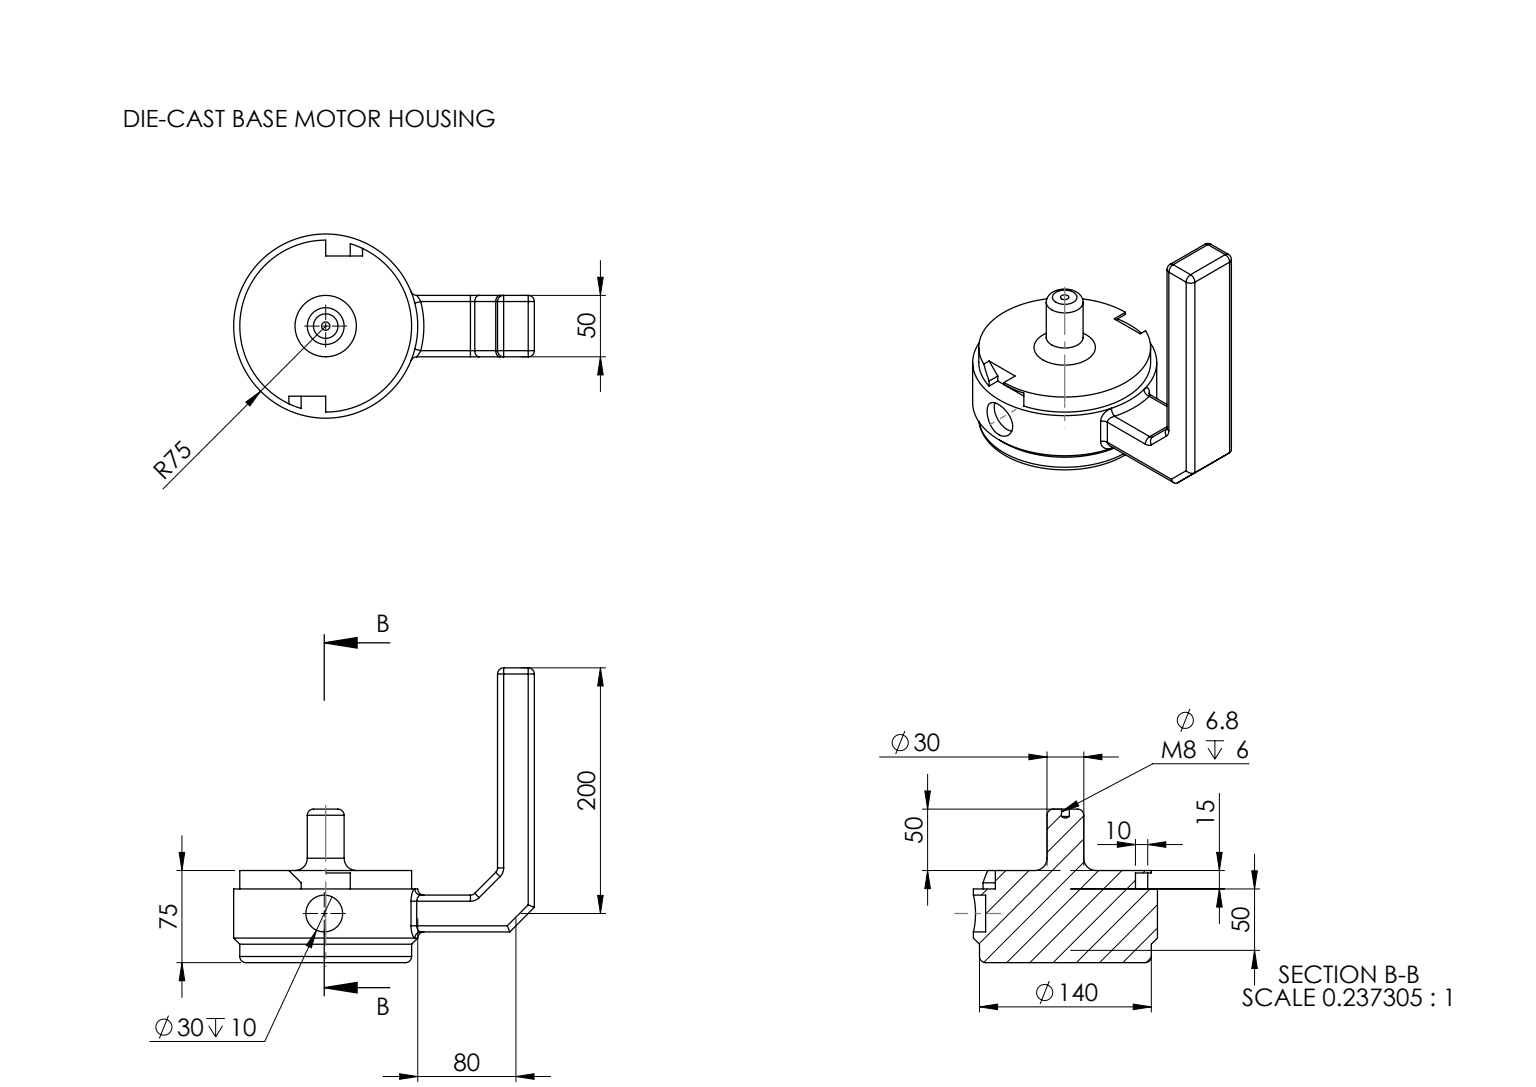
ISO-10303-21;
HEADER;
FILE_DESCRIPTION (('STEP AP214'),
    '1' );
FILE_NAME ('Die-Cast Base Motor Housing.step',
    '2026-10-08T14:59:03',
    ( '' ),
    ( '' ),
    'SwSTEP 2.0',
    'SolidWorks 2026',
    '' );
FILE_SCHEMA (( 'AUTOMOTIVE_DESIGN' ));
ENDSEC;

DATA;
#3=CARTESIAN_POINT ( 'NONE',  ( 71.93323519045090109, 49.64954395535312415, 21.22984507177767100 ) ) ;
#9=MECHANICAL_DESIGN_GEOMETRIC_PRESENTATION_REPRESENTATION('',(#5399),#3796);
#10=CARTESIAN_POINT ( 'NONE',  ( 1.836970198721029589E-15, 110.0000000000000000, 15.00000000000000000 ) ) ;
#18=CYLINDRICAL_SURFACE ( 'NONE', #1272, 5.000000000000001776 ) ;
#31=CARTESIAN_POINT ( 'NONE',  ( 74.19588822391826000, 40.66783446091307042, -24.95803700703555350 ) ) ;
#36=CARTESIAN_POINT ( 'NONE',  ( 77.29209776116614705, 15.00000000000009059, -20.32449628861697377 ) ) ;
#44=VERTEX_POINT ( 'NONE', #11902 ) ;
#50=CARTESIAN_POINT ( 'NONE',  ( 170.0000000000011369, 35.00000000000004974, -19.99999999999999645 ) ) ;
#51=VERTEX_POINT ( 'NONE', #2763 ) ;
#52=ADVANCED_FACE ( 'NONE', ( #8078 ), #12195, .T. ) ;
#53=PLANE ( 'NONE',  #708 ) ;
#58=VECTOR ( 'NONE', #5099, 1000.000000000000000 ) ;
#61=ADVANCED_FACE ( 'NONE', ( #9422 ), #904, .T. ) ;
#63=ADVANCED_FACE ( 'NONE', ( #7151 ), #4694, .T. ) ;
#64=CARTESIAN_POINT ( 'NONE',  ( -5.632982942078911925, 15.66369320862007264, 74.78974241430267966 ) ) ;
#75=CARTESIAN_POINT ( 'NONE',  ( 72.29554967163173274, 10.06394264408140771, 19.96827991394381030 ) ) ;
#79=AXIS2_PLACEMENT_3D ( 'NONE', #1491, #4293, #8024 ) ;
#81=CYLINDRICAL_SURFACE ( 'NONE', #3664, 5.000000000000000888 ) ;
#94=CARTESIAN_POINT ( 'NONE',  ( 74.77359728361332714, 42.68513822356444365, -24.22100760279283094 ) ) ;
#98=DIRECTION ( 'NONE',  ( 1.000000000000000000, 0.000000000000000000, -3.469446951953613203E-16 ) ) ;
#117=DIRECTION ( 'NONE',  ( 1.000000000000000000, -0.000000000000000000, 0.000000000000000000 ) ) ;
#121=ORIENTED_EDGE ( 'NONE', *, *, #6558, .F. ) ;
#123=DIRECTION ( 'NONE',  ( 1.000000000000000000, 0.000000000000000000, 0.000000000000000000 ) ) ;
#128=PLANE ( 'NONE',  #8446 ) ;
#131=DIRECTION ( 'NONE',  ( -1.000000000000000000, -1.387778780781444492E-15, 0.000000000000000000 ) ) ;
#134=CARTESIAN_POINT ( 'NONE',  ( 69.52686081652184669, 20.00000000000009237, -28.12499999999999645 ) ) ;
#137=CARTESIAN_POINT ( 'NONE',  ( 20.00000000000000000, 7.965803112215716020, -67.08203932499371547 ) ) ;
#141=ADVANCED_FACE ( 'NONE', ( #5767 ), #10055, .F. ) ;
#143=PLANE ( 'NONE',  #4255 ) ;
#149=DIRECTION ( 'NONE',  ( -0.000000000000000000, -0.000000000000000000, 1.000000000000000000 ) ) ;
#155=FILL_AREA_STYLE_COLOUR ( '', #11172 ) ;
#157=CARTESIAN_POINT ( 'NONE',  ( 70.81305327821827689, 40.84876555524851938, -24.93520811514266100 ) ) ;
#164=CARTESIAN_POINT ( 'NONE',  ( 76.56941542346943663, 15.25646994755911656, -21.58911091692574047 ) ) ;
#172=DIRECTION ( 'NONE',  ( 1.000000000000000000, 0.000000000000000000, 3.469446951953613203E-16 ) ) ;
#177=ORIENTED_EDGE ( 'NONE', *, *, #6032, .T. ) ;
#179=VECTOR ( 'NONE', #1966, 1000.000000000000000 ) ;
#192=ORIENTED_EDGE ( 'NONE', *, *, #11363, .T. ) ;
#194=CARTESIAN_POINT ( 'NONE',  ( 150.0000000000010800, 15.00000000000008882, 20.00000000000000000 ) ) ;
#201=CARTESIAN_POINT ( 'NONE',  ( 72.61843774138908714, 15.00000000000009059, 18.75000000000000355 ) ) ;
#202=CIRCLE ( 'NONE', #8371, 5.000000000000000888 ) ;
#203=ORIENTED_EDGE ( 'NONE', *, *, #11363, .F. ) ;
#206=VECTOR ( 'NONE', #5383, 1000.000000000000000 ) ;
#208=CARTESIAN_POINT ( 'NONE',  ( 13.11499952929491641, 34.60506461548092716, 73.84520852716261174 ) ) ;
#210=DIRECTION ( 'NONE',  ( -0.7071067811865503483, -0.7071067811865447972, -0.000000000000000000 ) ) ;
#211=DIRECTION ( 'NONE',  ( 0.000000000000000000, 1.000000000000000000, 0.000000000000000000 ) ) ;
#212=CARTESIAN_POINT ( 'NONE',  ( 0.000000000000000000, 10.00000000000017586, 0.000000000000000000 ) ) ;
#218=( LENGTH_UNIT ( ) NAMED_UNIT ( * ) SI_UNIT ( .MILLI., .METRE. ) );
#219=EDGE_CURVE ( 'NONE', #4313, #6757, #4559, .T. ) ;
#222=FACE_OUTER_BOUND ( 'NONE', #11804, .T. ) ;
#225=ADVANCED_FACE ( 'NONE', ( #3686 ), #6591, .F. ) ;
#229=CARTESIAN_POINT ( 'NONE',  ( 71.00672680945956472, 11.81742436800341345, -24.14780939829461204 ) ) ;
#234=AXIS2_PLACEMENT_3D ( 'NONE', #9468, #5745, #3808 ) ;
#250=VECTOR ( 'NONE', #7783, 1000.000000000000000 ) ;
#252=DIRECTION ( 'NONE',  ( -0.000000000000000000, 1.000000000000000000, -0.000000000000000000 ) ) ;
#254=CYLINDRICAL_SURFACE ( 'NONE', #5879, 5.000000000000000888 ) ;
#257=DIRECTION ( 'NONE',  ( -0.000000000000000000, -0.000000000000000000, 1.000000000000000000 ) ) ;
#261=CARTESIAN_POINT ( 'NONE',  ( -20.00000000000000000, 63.00000000000000000, -67.08203932499371547 ) ) ;
#270=CARTESIAN_POINT ( 'NONE',  ( 167.9289321881356614, 35.85786437626911294, 25.00000000000000000 ) ) ;
#273=CARTESIAN_POINT ( 'NONE',  ( 0.000000000000000000, 109.0000000000000000, 0.000000000000000000 ) ) ;
#276=DIRECTION ( 'NONE',  ( 0.000000000000000000, 1.000000000000000000, 0.000000000000000000 ) ) ;
#278=AXIS2_PLACEMENT_3D ( 'NONE', #5146, #9864, #5953 ) ;
#280=VECTOR ( 'NONE', #1354, 1000.000000000000000 ) ;
#282=ADVANCED_FACE ( 'NONE', ( #8294 ), #7374, .T. ) ;
#286=CYLINDRICAL_SURFACE ( 'NONE', #8857, 5.000000000000000888 ) ;
#287=CARTESIAN_POINT ( 'NONE',  ( 72.04420248082787737, 10.24880064609159724, -20.85013644286576096 ) ) ;
#288=CARTESIAN_POINT ( 'NONE',  ( 70.71657310242180472, 12.52464281459662310, -24.98455589012892375 ) ) ;
#294=CIRCLE ( 'NONE', #3880, 5.000000000000000888 ) ;
#298=VERTEX_POINT ( 'NONE', #8597 ) ;
#303=DIRECTION ( 'NONE',  ( 0.000000000000000000, -0.000000000000000000, 1.000000000000000000 ) ) ;
#305=CARTESIAN_POINT ( 'NONE',  ( 20.00000000000000355, 50.00000000000000000, -57.08203932499370836 ) ) ;
#309=AXIS2_PLACEMENT_3D ( 'NONE', #7223, #9134, #8895 ) ;
#312=ORIENTED_EDGE ( 'NONE', *, *, #4136, .T. ) ;
#314=CARTESIAN_POINT ( 'NONE',  ( 0.000000000000000000, 63.00000000000000000, 0.000000000000000000 ) ) ;
#317=PLANE ( 'NONE',  #6694 ) ;
#321=FACE_OUTER_BOUND ( 'NONE', #2192, .T. ) ;
#322=CARTESIAN_POINT ( 'NONE',  ( -30.00000000000004263, 65.00000000000000000, 57.08203932499370836 ) ) ;
#326=CARTESIAN_POINT ( 'NONE',  ( 72.18749622575050751, 14.85620204188371041, 20.39421446794931114 ) ) ;
#327=AXIS2_PLACEMENT_3D ( 'NONE', #339, #3397, #9993 ) ;
#328=ORIENTED_EDGE ( 'NONE', *, *, #7404, .T. ) ;
#329=CARTESIAN_POINT ( 'NONE',  ( 72.04250006633340320, 49.74972593579155244, -20.85600298363996430 ) ) ;
#333=CARTESIAN_POINT ( 'NONE',  ( 71.69683552452212894, 49.37956359449864863, 22.01474836615508579 ) ) ;
#335=CARTESIAN_POINT ( 'NONE',  ( 165.0000000000011369, 37.07106781186552524, -25.00000000000000000 ) ) ;
#339=CARTESIAN_POINT ( 'NONE',  ( 3.061616997868383043E-15, 75.00000000000000000, -25.00000000000000000 ) ) ;
#346=CARTESIAN_POINT ( 'NONE',  ( 0.000000000000000000, 115.0000000000000000, 0.000000000000000000 ) ) ;
#347=CARTESIAN_POINT ( 'NONE',  ( -30.00000000000004263, 65.00000000000000000, 63.24555320336758513 ) ) ;
#353=DIRECTION ( 'NONE',  ( 1.000000000000000000, -0.000000000000000000, 1.224646799147353207E-16 ) ) ;
#357=VERTEX_POINT ( 'NONE', #9483 ) ;
#364=DIRECTION ( 'NONE',  ( 0.000000000000000000, 0.000000000000000000, -1.000000000000000000 ) ) ;
#370=CARTESIAN_POINT ( 'NONE',  ( 0.000000000000000000, -10.00000000000000000, 0.000000000000000000 ) ) ;
#374=CARTESIAN_POINT ( 'NONE',  ( -20.00000000000000355, 50.00000000000000000, 57.08203932499370836 ) ) ;
#375=ORIENTED_EDGE ( 'NONE', *, *, #3119, .F. ) ;
#376=EDGE_CURVE ( 'NONE', #4020, #6378, #3189, .T. ) ;
#382=DIRECTION ( 'NONE',  ( -1.000000000000000000, 0.000000000000000000, -0.000000000000000000 ) ) ;
#383=CARTESIAN_POINT ( 'NONE',  ( 71.54629459846327677, 15.63701415187600219, 22.64784456521646661 ) ) ;
#390=CARTESIAN_POINT ( 'NONE',  ( 71.02603146012562263, 42.62559916300720175, -24.29862599233076637 ) ) ;
#391=ORIENTED_EDGE ( 'NONE', *, *, #7352, .F. ) ;
#393=CARTESIAN_POINT ( 'NONE',  ( 69.65901248891735520, 42.64626312845745559, 27.79625982057034150 ) ) ;
#400=DIRECTION ( 'NONE',  ( -1.000000000000000000, 0.000000000000000000, 2.213536252433181319E-16 ) ) ;
#404=AXIS2_PLACEMENT_3D ( 'NONE', #7515, #853, #5653 ) ;
#405=EDGE_CURVE ( 'NONE', #1040, #5376, #600, .T. ) ;
#406=CARTESIAN_POINT ( 'NONE',  ( 0.000000000000000000, -10.00000000000000000, -65.00000000000001421 ) ) ;
#436=FACE_OUTER_BOUND ( 'NONE', #4882, .T. ) ;
#437=CARTESIAN_POINT ( 'NONE',  ( 0.000000000000000000, 65.00000000000000000, 25.00000000000000000 ) ) ;
#443=DIRECTION ( 'NONE',  ( 0.000000000000000000, 0.000000000000000000, 1.000000000000000000 ) ) ;
#445=ORIENTED_EDGE ( 'NONE', *, *, #7746, .T. ) ;
#447=CARTESIAN_POINT ( 'NONE',  ( 74.19588822391826000, 19.33216553908705393, 24.95803700703554640 ) ) ;
#451=CARTESIAN_POINT ( 'NONE',  ( 74.19409830870891653, 19.27799416224737428, 24.96047248796920570 ) ) ;
#455=CARTESIAN_POINT ( 'NONE',  ( 70.92186449036606177, 47.98994378880887979, 24.39573567383822095 ) ) ;
#462=EDGE_LOOP ( 'NONE', ( #8985, #9947, #5228, #8018 ) ) ;
#466=CARTESIAN_POINT ( 'NONE',  ( 20.00000000000000355, 54.99999999999999289, -57.08203932499370836 ) ) ;
#472=CARTESIAN_POINT ( 'NONE',  ( 9.516722952433237737, 19.48499374783434845, 74.39444254373731269 ) ) ;
#477=ADVANCED_FACE ( 'NONE', ( #12331 ), #7566, .T. ) ;
#482=MANIFOLD_SOLID_BREP ( 'AdvancedHole1', #4496 ) ;
#484=CIRCLE ( 'NONE', #9229, 5.000000000000004441 ) ;
#487=ORIENTED_EDGE ( 'NONE', *, *, #800, .T. ) ;
#495=CARTESIAN_POINT ( 'NONE',  ( 71.93667174376723494, 49.65291573457426466, -21.21818801319906811 ) ) ;
#500=VECTOR ( 'NONE', #3071, 1000.000000000000000 ) ;
#511=CARTESIAN_POINT ( 'NONE',  ( 75.64991689405157160, 16.00507543303197266, 23.01117105493013781 ) ) ;
#512=CIRCLE ( 'NONE', #11671, 4.999999999999996447 ) ;
#515=ORIENTED_EDGE ( 'NONE', *, *, #3965, .F. ) ;
#520=CARTESIAN_POINT ( 'NONE',  ( 74.42783152987426831, 41.80108460718831509, 24.66728717810439875 ) ) ;
#521=ORIENTED_EDGE ( 'NONE', *, *, #9498, .F. ) ;
#528=EDGE_LOOP ( 'NONE', ( #1296, #3982, #5325, #5454 ) ) ;
#537=EDGE_CURVE ( 'NONE', #9081, #5052, #7524, .T. ) ;
#550=LINE ( 'NONE', #2356, #9259 ) ;
#552=CARTESIAN_POINT ( 'NONE',  ( 145.0000000000011369, 225.0000000000000853, 20.00000000000000000 ) ) ;
#555=CARTESIAN_POINT ( 'NONE',  ( 71.22480170918208842, 48.64519998125825140, -23.50133972577970809 ) ) ;
#560=DIRECTION ( 'NONE',  ( 0.000000000000000000, 1.000000000000000000, 0.000000000000000000 ) ) ;
#561=CARTESIAN_POINT ( 'NONE',  ( 20.00000000000000355, 50.00000000000000000, -57.08203932499370836 ) ) ;
#564=DIRECTION ( 'NONE',  ( 0.000000000000000000, 0.000000000000000000, -1.000000000000000000 ) ) ;
#565=LINE ( 'NONE', #4363, #10663 ) ;
#566=CIRCLE ( 'NONE', #6543, 5.000000000000000888 ) ;
#567=ORIENTED_EDGE ( 'NONE', *, *, #9997, .T. ) ;
#571=EDGE_LOOP ( 'NONE', ( #1015, #10303, #11033, #9480, #6919, #2706, #2009 ) ) ;
#573=CARTESIAN_POINT ( 'NONE',  ( 76.47547367680522257, 15.31088028275837232, 21.74308734404365850 ) ) ;
#575=ADVANCED_FACE ( 'NONE', ( #222 ), #10757, .T. ) ;
#576=CARTESIAN_POINT ( 'NONE',  ( 74.16198487095665826, 20.00000000000009237, 25.00000000000000000 ) ) ;
#580=CARTESIAN_POINT ( 'NONE',  ( 71.45054378765655656, 44.14136113826621255, 22.96278406504651315 ) ) ;
#582=EDGE_CURVE ( 'NONE', #2560, #3728, #10872, .T. ) ;
#587=TOROIDAL_SURFACE ( 'NONE', #2379, 9.999999999999998224, 5.000000000000000000 ) ;
#592=VERTEX_POINT ( 'NONE', #406 ) ;
#597=EDGE_CURVE ( 'NONE', #9722, #10814, #8003, .T. ) ;
#600=CIRCLE ( 'NONE', #5380, 9.999999999999994671 ) ;
#602=LINE ( 'NONE', #5341, #1517 ) ;
#604=CARTESIAN_POINT ( 'NONE',  ( 70.00771527461459698, 15.03038860802777776, -26.90815449096327328 ) ) ;
#609=EDGE_CURVE ( 'NONE', #5087, #6005, #11890, .T. ) ;
#615=ORIENTED_EDGE ( 'NONE', *, *, #10610, .F. ) ;
#628=ORIENTED_EDGE ( 'NONE', *, *, #8427, .T. ) ;
#642=AXIS2_PLACEMENT_3D ( 'NONE', #10504, #11452, #9314 ) ;
#644=ORIENTED_EDGE ( 'NONE', *, *, #7376, .F. ) ;
#646=CARTESIAN_POINT ( 'NONE',  ( 30.00000000000003908, 65.00000000000000000, -57.08203932499370836 ) ) ;
#648=FACE_OUTER_BOUND ( 'NONE', #3660, .T. ) ;
#649=DIRECTION ( 'NONE',  ( 0.000000000000000000, 1.000000000000000000, 0.000000000000000000 ) ) ;
#652=DIRECTION ( 'NONE',  ( 8.659560562354884787E-17, 0.7071067811865514585, -0.7071067811865435759 ) ) ;
#658=AXIS2_PLACEMENT_3D ( 'NONE', #9211, #5493, #5618 ) ;
#682=ORIENTED_EDGE ( 'NONE', *, *, #3384, .F. ) ;
#686=VERTEX_POINT ( 'NONE', #466 ) ;
#690=ORIENTED_EDGE ( 'NONE', *, *, #7585, .T. ) ;
#697=AXIS2_PLACEMENT_3D ( 'NONE', #6869, #3941, #4122 ) ;
#700=ADVANCED_FACE ( 'NONE', ( #5336 ), #7838, .T. ) ;
#708=AXIS2_PLACEMENT_3D ( 'NONE', #3868, #1310, #303 ) ;
#710=DIRECTION ( 'NONE',  ( 0.000000000000000000, 0.000000000000000000, 1.000000000000000000 ) ) ;
#711=CARTESIAN_POINT ( 'NONE',  ( 70.71067811865476926, 40.00000000000009237, 25.00000000000000000 ) ) ;
#712=VERTEX_POINT ( 'NONE', #10939 ) ;
#714=CARTESIAN_POINT ( 'NONE',  ( 74.16198487095665826, 50.00000000000000000, -30.00000000000000355 ) ) ;
#715=CARTESIAN_POINT ( 'NONE',  ( 72.54053945716880492, 45.08045300297751368, 19.05169875841045624 ) ) ;
#719=COLOUR_RGB ( '', 0.66274510, 0.83137255, 0.94901961) ;
#728=DIRECTION ( 'NONE',  ( 0.000000000000000000, 0.000000000000000000, -1.000000000000000000 ) ) ;
#730=CARTESIAN_POINT ( 'NONE',  ( 170.0000000000012221, 35.00000000000009948, -22.92893218813452805 ) ) ;
#735=CARTESIAN_POINT ( 'NONE',  ( -5.626974384805541796, 44.33833482606972609, 74.79022370185268187 ) ) ;
#736=CARTESIAN_POINT ( 'NONE',  ( 11.99712217873418574, 22.83768897326552505, 74.03455026502679459 ) ) ;
#737=VERTEX_POINT ( 'NONE', #6210 ) ;
#740=AXIS2_PLACEMENT_3D ( 'NONE', #9032, #11737, #443 ) ;
#746=ORIENTED_EDGE ( 'NONE', *, *, #1750, .F. ) ;
#752=DIRECTION ( 'NONE',  ( 0.000000000000000000, 0.000000000000000000, 1.000000000000000000 ) ) ;
#753=ORIENTED_EDGE ( 'NONE', *, *, #537, .T. ) ;
#767=AXIS2_PLACEMENT_3D ( 'NONE', #8094, #2433, #6238 ) ;
#787=ORIENTED_EDGE ( 'NONE', *, *, #9770, .F. ) ;
#788=DIRECTION ( 'NONE',  ( -0.7071067811865433539, 0.7071067811865517916, 0.000000000000000000 ) ) ;
#789=DIRECTION ( 'NONE',  ( -0.7071067811865495711, -0.7071067811865455743, -0.000000000000000000 ) ) ;
#790=CARTESIAN_POINT ( 'NONE',  ( 69.52686081652184669, 50.00000000000000000, -28.12500000000000000 ) ) ;
#794=CARTESIAN_POINT ( 'NONE',  ( 72.61843774138907293, 10.00000000000017586, 18.75000000000000000 ) ) ;
#800=EDGE_CURVE ( 'NONE', #51, #8715, #2709, .T. ) ;
#805=CARTESIAN_POINT ( 'NONE',  ( 74.16198487095664404, 20.00000000000008882, -24.99999999999999645 ) ) ;
#811=EDGE_LOOP ( 'NONE', ( #487, #3572, #7539, #8514, #12336, #11658, #7127 ) ) ;
#814=AXIS2_PLACEMENT_3D ( 'NONE', #8418, #12242, #891 ) ;
#818=ORIENTED_EDGE ( 'NONE', *, *, #6558, .T. ) ;
#819=ORIENTED_EDGE ( 'NONE', *, *, #9007, .T. ) ;
#823=LINE ( 'NONE', #3562, #4087 ) ;
#824=CIRCLE ( 'NONE', #8564, 5.000000000000000888 ) ;
#827=CARTESIAN_POINT ( 'NONE',  ( 145.0000000000011369, 225.0000000000000853, 20.00000000000000000 ) ) ;
#831=AXIS2_PLACEMENT_3D ( 'NONE', #8668, #7805, #6747 ) ;
#834=VERTEX_POINT ( 'NONE', #5771 ) ;
#838=CARTESIAN_POINT ( 'NONE',  ( 0.000000000000000000, 63.00000000000000000, 0.000000000000000000 ) ) ;
#841=FACE_OUTER_BOUND ( 'NONE', #9772, .T. ) ;
#845=CARTESIAN_POINT ( 'NONE',  ( 0.000000000000000000, 65.00000000000000000, 0.000000000000000000 ) ) ;
#846=ADVANCED_FACE ( 'NONE', ( #8558 ), #18, .T. ) ;
#847=ORIENTED_EDGE ( 'NONE', *, *, #11408, .T. ) ;
#849=DIRECTION ( 'NONE',  ( -0.000000000000000000, 1.000000000000000000, -0.000000000000000000 ) ) ;
#853=DIRECTION ( 'NONE',  ( 0.000000000000000000, 1.000000000000000000, 0.000000000000000000 ) ) ;
#854=EDGE_CURVE ( 'NONE', #5882, #9199, #10221, .T. ) ;
#856=DIRECTION ( 'NONE',  ( 0.000000000000000000, 0.000000000000000000, 1.000000000000000000 ) ) ;
#858=CIRCLE ( 'NONE', #2242, 5.000000000000000888 ) ;
#863=ADVANCED_FACE ( 'NONE', ( #8621 ), #81, .F. ) ;
#866=CARTESIAN_POINT ( 'NONE',  ( -20.00000000000000355, 7.965803112215716020, 57.08203932499370836 ) ) ;
#876=LINE ( 'NONE', #2799, #9503 ) ;
#877=DIRECTION ( 'NONE',  ( -3.469446951953613203E-16, 0.000000000000000000, 1.000000000000000000 ) ) ;
#890=ORIENTED_EDGE ( 'NONE', *, *, #376, .T. ) ;
#891=DIRECTION ( 'NONE',  ( 0.000000000000000000, 0.000000000000000000, 1.000000000000000000 ) ) ;
#892=CARTESIAN_POINT ( 'NONE',  ( 70.19857488179019356, 45.78302546620885494, 26.40439979598030718 ) ) ;
#895=CYLINDRICAL_SURFACE ( 'NONE', #7648, 5.000000000000000888 ) ;
#896=FACE_OUTER_BOUND ( 'NONE', #10777, .T. ) ;
#904=CYLINDRICAL_SURFACE ( 'NONE', #3502, 70.00000000000001421 ) ;
#905=AXIS2_PLACEMENT_3D ( 'NONE', #2605, #3666, #12028 ) ;
#908=ORIENTED_EDGE ( 'NONE', *, *, #9647, .F. ) ;
#918=ADVANCED_FACE ( 'NONE', ( #4896 ), #143, .F. ) ;
#923=CARTESIAN_POINT ( 'NONE',  ( 72.18749622575050751, 45.14379795811530727, -20.39421446795105197 ) ) ;
#924=VECTOR ( 'NONE', #4990, 1000.000000000000000 ) ;
#930=CARTESIAN_POINT ( 'NONE',  ( 69.62792625627730558, 17.67721533924630961, -27.87393767067208827 ) ) ;
#934=VERTEX_POINT ( 'NONE', #7755 ) ;
#937=EDGE_CURVE ( 'NONE', #2246, #11684, #2206, .T. ) ;
#942=AXIS2_PLACEMENT_3D ( 'NONE', #4143, #10750, #1402 ) ;
#958=ORIENTED_EDGE ( 'NONE', *, *, #6551, .T. ) ;
#963=DIRECTION ( 'NONE',  ( 0.000000000000000000, -1.000000000000000000, 0.000000000000000000 ) ) ;
#964=CARTESIAN_POINT ( 'NONE',  ( 145.0000000000011369, 67.07106781186550393, -20.00000000000000000 ) ) ;
#982=EDGE_CURVE ( 'NONE', #9665, #9072, #11640, .T. ) ;
#983=CARTESIAN_POINT ( 'NONE',  ( 71.13813068160534669, 43.14388772265235872, -23.95492789737679828 ) ) ;
#986=FACE_OUTER_BOUND ( 'NONE', #8799, .T. ) ;
#988=CARTESIAN_POINT ( 'NONE',  ( 75.64998878962165918, 16.00502810556076838, -23.01105902605769771 ) ) ;
#1002=ORIENTED_EDGE ( 'NONE', *, *, #219, .T. ) ;
#1006=FACE_OUTER_BOUND ( 'NONE', #3139, .T. ) ;
#1013=CARTESIAN_POINT ( 'NONE',  ( 0.000000000000000000, -5.000000000000000000, 0.000000000000000000 ) ) ;
#1014=CARTESIAN_POINT ( 'NONE',  ( -12.10445966455964673, 19.69657992720446060, 74.01758460308430188 ) ) ;
#1015=ORIENTED_EDGE ( 'NONE', *, *, #9080, .T. ) ;
#1016=DIRECTION ( 'NONE',  ( 0.000000000000000000, -1.000000000000000000, 0.000000000000000000 ) ) ;
#1017=CARTESIAN_POINT ( 'NONE',  ( 70.07436679451828354, 14.74552910246825199, 26.73229126030999581 ) ) ;
#1018=AXIS2_PLACEMENT_3D ( 'NONE', #6463, #8626, #10253 ) ;
#1019=ORIENTED_EDGE ( 'NONE', *, *, #8682, .F. ) ;
#1021=EDGE_CURVE ( 'NONE', #10899, #10965, #7929, .T. ) ;
#1027=AXIS2_PLACEMENT_3D ( 'NONE', #8343, #7711, #5908 ) ;
#1028=CARTESIAN_POINT ( 'NONE',  ( 77.29025109341935718, 15.00000000000008882, 20.32807234521490614 ) ) ;
#1029=EDGE_CURVE ( 'NONE', #6450, #6026, #6786, .T. ) ;
#1032=CARTESIAN_POINT ( 'NONE',  ( 13.37359372499693499, 33.71046439641005321, 73.79822922526992102 ) ) ;
#1035=CARTESIAN_POINT ( 'NONE',  ( -20.00000000000000355, 50.00000000000000000, 57.08203932499370836 ) ) ;
#1037=DIRECTION ( 'NONE',  ( 0.000000000000000000, 0.000000000000000000, 1.000000000000000000 ) ) ;
#1038=EDGE_LOOP ( 'NONE', ( #10956, #1512, #4611, #5247 ) ) ;
#1040=VERTEX_POINT ( 'NONE', #4378 ) ;
#1042=CARTESIAN_POINT ( 'NONE',  ( 69.92278643102426372, 44.50372822854298960, -27.12617897809110801 ) ) ;
#1052=EDGE_LOOP ( 'NONE', ( #3247, #9803, #3678, #1729 ) ) ;
#1057=CARTESIAN_POINT ( 'NONE',  ( 75.04216158314673635, 43.19040419545773091, 23.86402193374160774 ) ) ;
#1061=ADVANCED_FACE ( 'NONE', ( #648 ), #5386, .T. ) ;
#1063=EDGE_CURVE ( 'NONE', #5388, #11288, #3392, .T. ) ;
#1072=ORIENTED_EDGE ( 'NONE', *, *, #1029, .T. ) ;
#1074=FACE_OUTER_BOUND ( 'NONE', #4518, .T. ) ;
#1081=AXIS2_PLACEMENT_3D ( 'NONE', #8410, #2682, #2741 ) ;
#1087=CARTESIAN_POINT ( 'NONE',  ( 77.11525298301567943, 15.03197132203681363, 20.64974928742876159 ) ) ;
#1097=LINE ( 'NONE', #4901, #179 ) ;
#1104=ORIENTED_EDGE ( 'NONE', *, *, #6468, .T. ) ;
#1107=CARTESIAN_POINT ( 'NONE',  ( 71.43334412524781385, 49.01058866048808227, -22.86096127246359444 ) ) ;
#1111=CARTESIAN_POINT ( 'NONE',  ( 71.43628325305918736, 10.98492395331197358, -22.85167202658751151 ) ) ;
#1130=CIRCLE ( 'NONE', #1914, 75.00000000000001421 ) ;
#1139=CARTESIAN_POINT ( 'NONE',  ( 7.960204194457798830E-15, -5.000000000000000000, 65.00000000000001421 ) ) ;
#1140=CARTESIAN_POINT ( 'NONE',  ( -4.134262057974781968, 15.28257175693984848, 74.88765946342873292 ) ) ;
#1142=CARTESIAN_POINT ( 'NONE',  ( 0.000000000000000000, 10.00000000000009237, 0.000000000000000000 ) ) ;
#1144=ORIENTED_EDGE ( 'NONE', *, *, #10068, .T. ) ;
#1145=CARTESIAN_POINT ( 'NONE',  ( 0.000000000000000000, 63.00000000000000000, 0.000000000000000000 ) ) ;
#1150=CARTESIAN_POINT ( 'NONE',  ( 72.53968727264557970, 14.91866686485657922, 19.05499925486891755 ) ) ;
#1151=ADVANCED_FACE ( 'NONE', ( #7257 ), #11878, .F. ) ;
#1156=EDGE_LOOP ( 'NONE', ( #2013, #2025, #6086, #753 ) ) ;
#1163=CARTESIAN_POINT ( 'NONE',  ( 170.0000000000011369, 30.00000000000008882, 20.00000000000000000 ) ) ;
#1171=ORIENTED_EDGE ( 'NONE', *, *, #2583, .F. ) ;
#1173=CARTESIAN_POINT ( 'NONE',  ( 75.22303488722339182, 16.54275665089875247, -23.61575757524069630 ) ) ;
#1184=CARTESIAN_POINT ( 'NONE',  ( 74.31403689601796714, 41.40717934585230608, 24.81089180822486284 ) ) ;
#1188=ORIENTED_EDGE ( 'NONE', *, *, #2623, .T. ) ;
#1191=CARTESIAN_POINT ( 'NONE',  ( 20.00000000000000000, 50.00000000000000000, -67.08203932499371547 ) ) ;
#1198=CARTESIAN_POINT ( 'NONE',  ( -5.139633753169690955, 15.51989858384737531, 74.82538224130733795 ) ) ;
#1200=DIRECTION ( 'NONE',  ( 0.000000000000000000, 0.000000000000000000, 1.000000000000000000 ) ) ;
#1211=AXIS2_PLACEMENT_3D ( 'NONE', #1906, #1843, #856 ) ;
#1217=CARTESIAN_POINT ( 'NONE',  ( 4.520246555170921887, 43.87820047625252329, 74.86495189574776532 ) ) ;
#1220=FACE_OUTER_BOUND ( 'NONE', #8472, .T. ) ;
#1221=DIRECTION ( 'NONE',  ( 0.000000000000000000, 0.000000000000000000, -1.000000000000000000 ) ) ;
#1228=AXIS2_PLACEMENT_3D ( 'NONE', #11079, #4530, #5225 ) ;
#1231=VERTEX_POINT ( 'NONE', #3634 ) ;
#1233=CARTESIAN_POINT ( 'NONE',  ( 71.26309188267669015, 11.28349307498528020, -23.38502809576078079 ) ) ;
#1234=CARTESIAN_POINT ( 'NONE',  ( 70.96538090731310433, 11.90979482576331883, -24.26905913879961929 ) ) ;
#1242=ADVANCED_FACE ( 'NONE', ( #12247 ), #895, .T. ) ;
#1244=VERTEX_POINT ( 'NONE', #11309 ) ;
#1245=CARTESIAN_POINT ( 'NONE',  ( 0.000000000000000000, 65.00000000000000000, 0.000000000000000000 ) ) ;
#1249=CARTESIAN_POINT ( 'NONE',  ( 2.020667218593133416E-14, 65.00000000000000000, 70.00000000000000000 ) ) ;
#1269=CARTESIAN_POINT ( 'NONE',  ( 71.40110041870237012, 15.97341095676601697, 23.12535642331794605 ) ) ;
#1272=AXIS2_PLACEMENT_3D ( 'NONE', #6702, #7511, #788 ) ;
#1281=FACE_OUTER_BOUND ( 'NONE', #7568, .T. ) ;
#1283=DIRECTION ( 'NONE',  ( 0.000000000000000000, 1.000000000000000000, 0.000000000000000000 ) ) ;
#1289=DIRECTION ( 'NONE',  ( -0.2499999999999996947, 0.000000000000000000, -0.9682458365518543664 ) ) ;
#1290=DIRECTION ( 'NONE',  ( 0.000000000000000000, 0.000000000000000000, 1.000000000000000000 ) ) ;
#1296=ORIENTED_EDGE ( 'NONE', *, *, #10352, .T. ) ;
#1302=ADVANCED_FACE ( 'NONE', ( #6689 ), #4871, .F. ) ;
#1306=DIRECTION ( 'NONE',  ( -0.000000000000000000, -1.000000000000000000, -0.000000000000000000 ) ) ;
#1310=DIRECTION ( 'NONE',  ( 0.000000000000000000, 1.000000000000000000, 0.000000000000000000 ) ) ;
#1316=VECTOR ( 'NONE', #3519, 1000.000000000000000 ) ;
#1319=DIRECTION ( 'NONE',  ( 0.000000000000000000, 0.000000000000000000, 1.000000000000000000 ) ) ;
#1327=CARTESIAN_POINT ( 'NONE',  ( 121.4644660940682428, 46.46446609406732620, -20.00000000000000000 ) ) ;
#1329=CARTESIAN_POINT ( 'NONE',  ( 165.0000000000011369, 225.0000000000000853, -20.00000000000000000 ) ) ;
#1331=CARTESIAN_POINT ( 'NONE',  ( 71.99568681135517068, 14.96114988300740656, 21.09760594592229310 ) ) ;
#1333=EDGE_CURVE ( 'NONE', #11288, #6005, #8038, .T. ) ;
#1336=CARTESIAN_POINT ( 'NONE',  ( 70.79540202493410561, 40.42529689935005877, -24.98706380095369894 ) ) ;
#1339=CARTESIAN_POINT ( 'NONE',  ( 71.78382695943244585, 49.48706010510388609, 21.72958296927689759 ) ) ;
#1344=CARTESIAN_POINT ( 'NONE',  ( 0.000000000000000000, 110.0000000000000000, 0.000000000000000000 ) ) ;
#1352=DIRECTION ( 'NONE',  ( 0.000000000000000000, 1.000000000000000000, -0.000000000000000000 ) ) ;
#1353=CARTESIAN_POINT ( 'NONE',  ( -0.5177535225088374382, 44.99389217799025431, 75.00000000000001421 ) ) ;
#1354=DIRECTION ( 'NONE',  ( 0.000000000000000000, 1.000000000000000000, 0.000000000000000000 ) ) ;
#1356=ORIENTED_EDGE ( 'NONE', *, *, #7015, .F. ) ;
#1363=EDGE_LOOP ( 'NONE', ( #3842, #1356, #12095, #9800 ) ) ;
#1365=PLANE ( 'NONE',  #6497 ) ;
#1366=ORIENTED_EDGE ( 'NONE', *, *, #8545, .T. ) ;
#1367=DIRECTION ( 'NONE',  ( 1.000000000000000000, -0.000000000000000000, 0.000000000000000000 ) ) ;
#1373=CARTESIAN_POINT ( 'NONE',  ( 70.40708232491709850, 46.56656424045070253, -25.84664880093518136 ) ) ;
#1375=CARTESIAN_POINT ( 'NONE',  ( 1.734723475976807094E-14, 65.00000000000000000, 57.08203932499370836 ) ) ;
#1376=CARTESIAN_POINT ( 'NONE',  ( 125.0000000000009663, 42.92893218813457423, 20.00000000000000000 ) ) ;
#1378=ORIENTED_EDGE ( 'NONE', *, *, #3887, .F. ) ;
#1379=DIRECTION ( 'NONE',  ( 1.000000000000000000, 0.000000000000000000, 0.000000000000000000 ) ) ;
#1382=DIRECTION ( 'NONE',  ( 3.469446951953613203E-16, 0.000000000000000000, -1.000000000000000000 ) ) ;
#1383=CARTESIAN_POINT ( 'NONE',  ( 74.31677170407374433, 41.41979450890040937, -24.80746953044373981 ) ) ;
#1384=CARTESIAN_POINT ( 'NONE',  ( 74.16198487095664404, 40.00000000000009237, 29.99999999999999645 ) ) ;
#1387=CARTESIAN_POINT ( 'NONE',  ( 69.57792926911190534, 18.32862386349516015, 27.99850680361992517 ) ) ;
#1388=CIRCLE ( 'NONE', #8934, 5.000000000000000888 ) ;
#1390=EDGE_LOOP ( 'NONE', ( #3549, #192, #5200, #5928 ) ) ;
#1391=CARTESIAN_POINT ( 'NONE',  ( 72.28000013808933488, 45.16202677360365669, -20.04822706562131884 ) ) ;
#1394=ADVANCED_FACE ( 'NONE', ( #3128 ), #9173, .T. ) ;
#1397=CARTESIAN_POINT ( 'NONE',  ( 75.14265900998388759, 43.33802077090974336, 23.72616954495132191 ) ) ;
#1400=AXIS2_PLACEMENT_3D ( 'NONE', #6661, #1798, #8459 ) ;
#1402=DIRECTION ( 'NONE',  ( 0.000000000000000000, 0.000000000000000000, 1.000000000000000000 ) ) ;
#1404=ADVANCED_FACE ( 'NONE', ( #2247 ), #2946, .T. ) ;
#1407=ORIENTED_EDGE ( 'NONE', *, *, #9808, .F. ) ;
#1418=CARTESIAN_POINT ( 'NONE',  ( 71.22405252493085470, 11.35584875400091320, -23.50371070993386624 ) ) ;
#1428=CARTESIAN_POINT ( 'NONE',  ( 74.31403689601799556, 18.59282065414787510, -24.81089180822486639 ) ) ;
#1447=DIRECTION ( 'NONE',  ( -0.000000000000000000, 1.000000000000000000, -0.000000000000000000 ) ) ;
#1452=CARTESIAN_POINT ( 'NONE',  ( 74.77359728361332714, 17.31486177643626334, 24.22100760279318621 ) ) ;
#1455=CARTESIAN_POINT ( 'NONE',  ( 72.29554967163204537, 49.93605735591993522, -19.96827991394273383 ) ) ;
#1460=CARTESIAN_POINT ( 'NONE',  ( 74.38206444891756064, 41.64350558143038228, 24.72514820121040557 ) ) ;
#1461=AXIS2_PLACEMENT_3D ( 'NONE', #1376, #1564, #4301 ) ;
#1467=EDGE_LOOP ( 'NONE', ( #12126, #5840 ) ) ;
#1480=CARTESIAN_POINT ( 'NONE',  ( 8.572527594031472993E-15, 63.00000000000000000, -70.00000000000000000 ) ) ;
#1483=ADVANCED_FACE ( 'NONE', ( #11922 ), #11863, .F. ) ;
#1484=AXIS2_PLACEMENT_3D ( 'NONE', #3606, #1556, #5359 ) ;
#1489=FACE_OUTER_BOUND ( 'NONE', #2859, .T. ) ;
#1491=CARTESIAN_POINT ( 'NONE',  ( 165.0000000000011369, 30.00000000000008882, -19.99999999999999645 ) ) ;
#1498=EDGE_CURVE ( 'NONE', #5994, #10814, #4603, .T. ) ;
#1501=DIRECTION ( 'NONE',  ( -0.000000000000000000, 1.000000000000000000, -0.000000000000000000 ) ) ;
#1512=ORIENTED_EDGE ( 'NONE', *, *, #8707, .F. ) ;
#1514=CARTESIAN_POINT ( 'NONE',  ( 75.13748311126856549, 16.66004759637138832, 23.73500236558975729 ) ) ;
#1515=ADVANCED_FACE ( 'NONE', ( #5310 ), #6119, .F. ) ;
#1517=VECTOR ( 'NONE', #3348, 1000.000000000000000 ) ;
#1519=CARTESIAN_POINT ( 'NONE',  ( 72.61843774138908714, 50.00000000000009237, -18.75000000000000355 ) ) ;
#1524=CARTESIAN_POINT ( 'NONE',  ( 76.01396467472481788, 44.35825346231943200, 22.47201498426101196 ) ) ;
#1530=ADVANCED_FACE ( 'NONE', ( #7304 ), #7973, .T. ) ;
#1531=ORIENTED_EDGE ( 'NONE', *, *, #9964, .T. ) ;
#1543=CARTESIAN_POINT ( 'NONE',  ( 69.55111042745876659, 18.70063303202293170, -28.06526308249821966 ) ) ;
#1555=EDGE_LOOP ( 'NONE', ( #9556, #567, #3671, #10469, #7819, #2628, #1688, #11556, #2618, #8107 ) ) ;
#1556=DIRECTION ( 'NONE',  ( 0.7071067811865495711, 0.7071067811865455743, 0.000000000000000000 ) ) ;
#1560=CARTESIAN_POINT ( 'NONE',  ( 69.55717041450675708, 41.30413405089374379, -28.04997484771492822 ) ) ;
#1563=CARTESIAN_POINT ( 'NONE',  ( -1.190781129305471087, 30.00000000000008882, 65.00000000000000000 ) ) ;
#1564=DIRECTION ( 'NONE',  ( -0.7071067811865503483, -0.7071067811865447972, 0.000000000000000000 ) ) ;
#1572=CARTESIAN_POINT ( 'NONE',  ( -20.00000000000000000, 50.00000000000000000, -67.08203932499371547 ) ) ;
#1573=DIRECTION ( 'NONE',  ( 0.000000000000000000, 0.000000000000000000, -1.000000000000000000 ) ) ;
#1578=DIRECTION ( 'NONE',  ( 3.469446951953613203E-16, 0.000000000000000000, 1.000000000000000000 ) ) ;
#1582=CARTESIAN_POINT ( 'NONE',  ( 74.70253266892970601, 42.54723899285758648, 24.31510929947630117 ) ) ;
#1589=CIRCLE ( 'NONE', #8536, 5.000000000000004441 ) ;
#1596=DIRECTION ( 'NONE',  ( -1.000000000000000000, -6.938893903907232322E-16, 0.000000000000000000 ) ) ;
#1602=CARTESIAN_POINT ( 'NONE',  ( 13.37325603157604270, 26.28968282453032757, 73.79828864025962787 ) ) ;
#1608=CARTESIAN_POINT ( 'NONE',  ( 4.953755887175457673, 16.30827223463906250, 74.83741081793274930 ) ) ;
#1612=AXIS2_PLACEMENT_3D ( 'NONE', #9562, #7823, #5032 ) ;
#1622=EDGE_CURVE ( 'NONE', #9381, #8789, #11980, .T. ) ;
#1624=B_SPLINE_CURVE_WITH_KNOTS ( 'NONE', 3,
 ( #9881, #1353, #5162, #6462, #1727, #3534, #8438, #735, #11270, #6528, #7336, #10313, #10252, #5655, #3471, #8317, #6581, #10122, #9374, #7401, #5533, #9312, #11078, #11136, #9250 ),
 .UNSPECIFIED., .F., .F.,
 ( 4, 2, 1, 2, 2, 2, 2, 2, 2, 2, 2, 2, 4 ),
 ( 0.04461974739530318729, 0.04616436123732098329, 0.04770897507933878623, 0.04925358892135658917, 0.05079820276337438517, 0.05388743044740997717, 0.05543204428942777318, 0.05697665813144557612, 0.06006588581548116812, 0.06315511349951676012, 0.06469972734153456306, 0.06624434118355236600, 0.06933356886758795801 ),
 .UNSPECIFIED. ) ;
#1629=PLANE ( 'NONE',  #7686 ) ;
#1633=CARTESIAN_POINT ( 'NONE',  ( 75.00000000000001421, 45.00000000000008527, -19.99999999999999645 ) ) ;
#1634=CARTESIAN_POINT ( 'NONE',  ( 0.000000000000000000, 75.00000000000000000, -15.00000000000000000 ) ) ;
#1646=CARTESIAN_POINT ( 'NONE',  ( 76.56941542346943663, 44.74353005244127246, 21.58911091692504769 ) ) ;
#1656=CARTESIAN_POINT ( 'NONE',  ( 165.0000000000011369, 230.0000000000000853, -25.00000000000000000 ) ) ;
#1666=DIRECTION ( 'NONE',  ( -0.7071067811865511255, -0.7071067811865440200, -0.000000000000000000 ) ) ;
#1673=EDGE_CURVE ( 'NONE', #10742, #4428, #2219, .T. ) ;
#1682=AXIS2_PLACEMENT_3D ( 'NONE', #1142, #6873, #1200 ) ;
#1684=ORIENTED_EDGE ( 'NONE', *, *, #1333, .F. ) ;
#1688=ORIENTED_EDGE ( 'NONE', *, *, #9305, .T. ) ;
#1693=AXIS2_PLACEMENT_3D ( 'NONE', #10136, #8329, #3602 ) ;
#1698=DIRECTION ( 'NONE',  ( 0.000000000000000000, 0.000000000000000000, 1.000000000000000000 ) ) ;
#1706=CARTESIAN_POINT ( 'NONE',  ( 70.40913241174638415, 46.55333156353304958, 25.83788073351891512 ) ) ;
#1707=ORIENTED_EDGE ( 'NONE', *, *, #3947, .T. ) ;
#1709=CARTESIAN_POINT ( 'NONE',  ( 72.29800075079560884, 49.93741478214614204, 19.95946618966863895 ) ) ;
#1710=ORIENTED_EDGE ( 'NONE', *, *, #12207, .T. ) ;
#1712=DIRECTION ( 'NONE',  ( 0.000000000000000000, 0.000000000000000000, -1.000000000000000000 ) ) ;
#1714=CIRCLE ( 'NONE', #4900, 70.00000000000000000 ) ;
#1716=ADVANCED_FACE ( 'NONE', ( #986 ), #6775, .F. ) ;
#1717=EDGE_LOOP ( 'NONE', ( #4444, #3307, #11764, #9702 ) ) ;
#1727=CARTESIAN_POINT ( 'NONE',  ( -3.103867246957984438, 44.90412228795011629, 74.94096782355340736 ) ) ;
#1728=CYLINDRICAL_SURFACE ( 'NONE', #642, 15.00000000000000000 ) ;
#1729=ORIENTED_EDGE ( 'NONE', *, *, #2791, .T. ) ;
#1731=CARTESIAN_POINT ( 'NONE',  ( -20.00000000000000355, 54.99999999999999289, 57.08203932499370836 ) ) ;
#1737=FACE_OUTER_BOUND ( 'NONE', #11293, .T. ) ;
#1747=VERTEX_POINT ( 'NONE', #7649 ) ;
#1749=ORIENTED_EDGE ( 'NONE', *, *, #3284, .F. ) ;
#1750=EDGE_CURVE ( 'NONE', #1040, #11448, #2977, .T. ) ;
#1753=LINE ( 'NONE', #1633, #4857 ) ;
#1763=CARTESIAN_POINT ( 'NONE',  ( 71.22405252493085470, 48.64415124599927509, 23.50371070993386269 ) ) ;
#1766=CARTESIAN_POINT ( 'NONE',  ( 72.61843774138908714, 50.00000000000009237, 18.75000000000001421 ) ) ;
#1769=CARTESIAN_POINT ( 'NONE',  ( 20.00000000000000355, 54.99999999999999289, -57.08203932499370836 ) ) ;
#1782=DIRECTION ( 'NONE',  ( 0.000000000000000000, 0.000000000000000000, 1.000000000000000000 ) ) ;
#1787=CARTESIAN_POINT ( 'NONE',  ( 8.125438539539757699, 18.23465150910980626, 74.55949004007592862 ) ) ;
#1791=FACE_OUTER_BOUND ( 'NONE', #528, .T. ) ;
#1798=DIRECTION ( 'NONE',  ( 0.000000000000000000, 1.000000000000000000, 0.000000000000000000 ) ) ;
#1802=TOROIDAL_SURFACE ( 'NONE', #2175, 25.00000000000000000, 10.00000000000000000 ) ;
#1815=CARTESIAN_POINT ( 'NONE',  ( 140.0000000000011369, 30.00000000000008882, -19.99999999999999645 ) ) ;
#1818=DIRECTION ( 'NONE',  ( -0.000000000000000000, 1.000000000000000000, -0.000000000000000000 ) ) ;
#1824=CARTESIAN_POINT ( 'NONE',  ( 70.96538090731311854, 48.09020517423687124, 24.26905913879962640 ) ) ;
#1843=DIRECTION ( 'NONE',  ( 0.000000000000000000, 1.000000000000000000, 0.000000000000000000 ) ) ;
#1846=CIRCLE ( 'NONE', #6229, 75.00000000000001421 ) ;
#1847=CARTESIAN_POINT ( 'NONE',  ( 70.29663099721912545, 46.18241670634586171, -26.14423569115638912 ) ) ;
#1856=ADVANCED_FACE ( 'NONE', ( #6960 ), #11895, .F. ) ;
#1857=CARTESIAN_POINT ( 'NONE',  ( 0.000000000000000000, 110.0000000000000000, 0.000000000000000000 ) ) ;
#1860=CIRCLE ( 'NONE', #3464, 5.000000000000004441 ) ;
#1861=EDGE_LOOP ( 'NONE', ( #5108, #9215, #11311, #11794 ) ) ;
#1864=EDGE_LOOP ( 'NONE', ( #10104, #8786, #1366, #11017 ) ) ;
#1868=CARTESIAN_POINT ( 'NONE',  ( 120.0000000000009948, 45.00000000000008527, 20.00000000000000000 ) ) ;
#1870=FACE_OUTER_BOUND ( 'NONE', #9953, .T. ) ;
#1880=CARTESIAN_POINT ( 'NONE',  ( 69.52686081652184669, 40.00000000000009237, 28.12499999999999645 ) ) ;
#1888=DIRECTION ( 'NONE',  ( -1.000000000000000000, 0.000000000000000000, 0.000000000000000000 ) ) ;
#1890=VECTOR ( 'NONE', #2398, 1000.000000000000000 ) ;
#1891=EDGE_CURVE ( 'NONE', #10740, #686, #5100, .T. ) ;
#1892=EDGE_CURVE ( 'NONE', #10506, #10768, #7516, .T. ) ;
#1893=DIRECTION ( 'NONE',  ( 0.000000000000000000, 0.000000000000000000, -1.000000000000000000 ) ) ;
#1901=CARTESIAN_POINT ( 'NONE',  ( 74.16198487095665826, 20.00000000000009237, -25.00000000000000000 ) ) ;
#1905=DIRECTION ( 'NONE',  ( 0.000000000000000000, 0.000000000000000000, 1.000000000000000000 ) ) ;
#1906=CARTESIAN_POINT ( 'NONE',  ( 0.000000000000000000, 50.00000000000000000, 0.000000000000000000 ) ) ;
#1910=( NAMED_UNIT ( * ) SI_UNIT ( $, .STERADIAN. ) SOLID_ANGLE_UNIT ( ) );
#1913=CARTESIAN_POINT ( 'NONE',  ( 75.64991689405155739, 43.99492456696821563, -23.01117105493013781 ) ) ;
#1914=AXIS2_PLACEMENT_3D ( 'NONE', #4529, #10376, #4585 ) ;
#1915=SURFACE_SIDE_STYLE ('',( #7709 ) ) ;
#1925=CIRCLE ( 'NONE', #5120, 65.00000000000001421 ) ;
#1934=DIRECTION ( 'NONE',  ( -1.000000000000000000, -0.000000000000000000, -0.000000000000000000 ) ) ;
#1945=CARTESIAN_POINT ( 'NONE',  ( 140.0000000000011369, 67.07106781186550393, 20.00000000000000000 ) ) ;
#1946=CARTESIAN_POINT ( 'NONE',  ( 20.00000000000000355, 50.00000000000000000, 57.08203932499370836 ) ) ;
#1949=CARTESIAN_POINT ( 'NONE',  ( 170.0000000000011369, 225.0000000000000853, 20.00000000000000000 ) ) ;
#1950=ORIENTED_EDGE ( 'NONE', *, *, #7796, .F. ) ;
#1951=CARTESIAN_POINT ( 'NONE',  ( 0.000000000000000000, 5.000000000000129674, 70.00000000000001421 ) ) ;
#1956=ORIENTED_EDGE ( 'NONE', *, *, #11945, .T. ) ;
#1962=CARTESIAN_POINT ( 'NONE',  ( 1.734723475976807094E-14, 63.00000000000000000, 57.08203932499370836 ) ) ;
#1966=DIRECTION ( 'NONE',  ( 0.000000000000000000, 1.000000000000000000, 0.000000000000000000 ) ) ;
#1967=CARTESIAN_POINT ( 'NONE',  ( 69.52686081652184669, 50.00000000000000000, 28.12500000000000000 ) ) ;
#1974=CARTESIAN_POINT ( 'NONE',  ( 70.67517779188629845, 47.36270866767235077, -25.10124566575549210 ) ) ;
#1976=CARTESIAN_POINT ( 'NONE',  ( 0.000000000000000000, 75.00000000000000000, 0.000000000000000000 ) ) ;
#1978=CARTESIAN_POINT ( 'NONE',  ( 70.23094937779806912, 14.08906915838008089, -26.31821466697866185 ) ) ;
#1989=ORIENTED_EDGE ( 'NONE', *, *, #5014, .F. ) ;
#1991=CARTESIAN_POINT ( 'NONE',  ( 74.40419232661420779, 41.74530093123432550, 24.69784343973813634 ) ) ;
#1998=DIRECTION ( 'NONE',  ( -3.469446951953619119E-16, 0.000000000000000000, -1.000000000000000000 ) ) ;
#2008=CARTESIAN_POINT ( 'NONE',  ( 0.000000000000000000, 50.00000000000000000, 0.000000000000000000 ) ) ;
#2009=ORIENTED_EDGE ( 'NONE', *, *, #9960, .T. ) ;
#2012=AXIS2_PLACEMENT_3D ( 'NONE', #1769, #2701, #3696 ) ;
#2013=ORIENTED_EDGE ( 'NONE', *, *, #11200, .T. ) ;
#2015=CARTESIAN_POINT ( 'NONE',  ( -20.00000000000004263, 7.965803112215716020, 67.08203932499370126 ) ) ;
#2025=ORIENTED_EDGE ( 'NONE', *, *, #11728, .T. ) ;
#2026=DIRECTION ( 'NONE',  ( -0.000000000000000000, 1.000000000000000000, -0.000000000000000000 ) ) ;
#2027=CARTESIAN_POINT ( 'NONE',  ( 6.210137148270883145, 43.08033144994158903, 74.74717517330344663 ) ) ;
#2030=PLANE ( 'NONE',  #7218 ) ;
#2031=DIRECTION ( 'NONE',  ( 1.000000000000000000, -0.000000000000000000, 0.000000000000000000 ) ) ;
#2039=CARTESIAN_POINT ( 'NONE',  ( 71.00573438501002954, 48.18030900481924306, -24.15070487907424734 ) ) ;
#2042=DIRECTION ( 'NONE',  ( 0.7071067811865513475, 0.7071067811865437980, -0.000000000000000000 ) ) ;
#2043=CARTESIAN_POINT ( 'NONE',  ( 72.61843774138908714, 10.00000000000009059, -18.74999999999999289 ) ) ;
#2044=ORIENTED_EDGE ( 'NONE', *, *, #4713, .T. ) ;
#2050=EDGE_CURVE ( 'NONE', #6378, #11448, #6157, .T. ) ;
#2052=AXIS2_PLACEMENT_3D ( 'NONE', #2556, #3243, #9968 ) ;
#2056=DIRECTION ( 'NONE',  ( 0.000000000000000000, 1.000000000000000000, 0.000000000000000000 ) ) ;
#2057=FACE_OUTER_BOUND ( 'NONE', #5797, .T. ) ;
#2063=ADVANCED_FACE ( 'NONE', ( #3962 ), #8562, .T. ) ;
#2069=SPHERICAL_SURFACE ( 'NONE', #9040, 5.000000000000000000 ) ;
#2074=VECTOR ( 'NONE', #3021, 1000.000000000000000 ) ;
#2078=DIRECTION ( 'NONE',  ( -3.469446951953613203E-16, 0.000000000000000000, -1.000000000000000000 ) ) ;
#2086=CARTESIAN_POINT ( 'NONE',  ( 117.9289321881355193, 45.00000000000008527, 25.00000000000000000 ) ) ;
#2087=EDGE_CURVE ( 'NONE', #11761, #6384, #7576, .T. ) ;
#2090=DIRECTION ( 'NONE',  ( 0.000000000000000000, -0.000000000000000000, 1.000000000000000000 ) ) ;
#2092=DIRECTION ( 'NONE',  ( 0.000000000000000000, 1.000000000000000000, 0.000000000000000000 ) ) ;
#2100=( NAMED_UNIT ( * ) SI_UNIT ( $, .STERADIAN. ) SOLID_ANGLE_UNIT ( ) );
#2102=VECTOR ( 'NONE', #7528, 1000.000000000000000 ) ;
#2107=CARTESIAN_POINT ( 'NONE',  ( 70.52159520668648440, 13.08551330184377370, -25.52954545350316451 ) ) ;
#2112=AXIS2_PLACEMENT_3D ( 'NONE', #7503, #649, #5637 ) ;
#2122=ORIENTED_EDGE ( 'NONE', *, *, #2843, .F. ) ;
#2123=EDGE_CURVE ( 'NONE', #10790, #5372, #4591, .T. ) ;
#2133=CARTESIAN_POINT ( 'NONE',  ( -13.10975425465743172, 20.87853446539744340, 73.84596017914877564 ) ) ;
#2137=ORIENTED_EDGE ( 'NONE', *, *, #3757, .F. ) ;
#2139=DIRECTION ( 'NONE',  ( -0.000000000000000000, 1.000000000000000000, -0.000000000000000000 ) ) ;
#2144=ORIENTED_EDGE ( 'NONE', *, *, #8075, .T. ) ;
#2148=ORIENTED_EDGE ( 'NONE', *, *, #2426, .F. ) ;
#2149=CARTESIAN_POINT ( 'NONE',  ( 150.0000000000010800, 15.00000000000008882, 25.00000000000000000 ) ) ;
#2154=ORIENTED_EDGE ( 'NONE', *, *, #8061, .T. ) ;
#2155=( NAMED_UNIT ( * ) PLANE_ANGLE_UNIT ( ) SI_UNIT ( $, .RADIAN. ) );
#2165=CARTESIAN_POINT ( 'NONE',  ( 72.18749001408211541, 14.85617579097899288, -20.39424303846762498 ) ) ;
#2171=DIRECTION ( 'NONE',  ( 3.469446951953613203E-16, 0.000000000000000000, -1.000000000000000000 ) ) ;
#2175=AXIS2_PLACEMENT_3D ( 'NONE', #10101, #6379, #710 ) ;
#2176=CARTESIAN_POINT ( 'NONE',  ( 0.000000000000000000, 225.0000000000000853, -20.00000000000000000 ) ) ;
#2181=EDGE_CURVE ( 'NONE', #3552, #3229, #1097, .T. ) ;
#2189=AXIS2_PLACEMENT_3D ( 'NONE', #11175, #10227, #123 ) ;
#2191=CARTESIAN_POINT ( 'NONE',  ( 71.66825662749600667, 10.65753464538973994, 22.10769995529666332 ) ) ;
#2192=EDGE_LOOP ( 'NONE', ( #7675, #746, #11330, #2503 ) ) ;
#2194=CARTESIAN_POINT ( 'NONE',  ( 74.75803814165917061, 42.66597992467871592, -24.24257051231691307 ) ) ;
#2200=TOROIDAL_SURFACE ( 'NONE', #2603, 9.999999999999998224, 5.000000000000000000 ) ;
#2202=CARTESIAN_POINT ( 'NONE',  ( 76.77549258727734127, 15.14783244007807994, 21.24643021050508551 ) ) ;
#2206=LINE ( 'NONE', #11633, #2074 ) ;
#2212=CARTESIAN_POINT ( 'NONE',  ( 145.0000000000011369, 0.000000000000000000, -25.00000000000000000 ) ) ;
#2219=CIRCLE ( 'NONE', #3217, 4.999999999999998224 ) ;
#2230=ORIENTED_EDGE ( 'NONE', *, *, #8427, .F. ) ;
#2234=DIRECTION ( 'NONE',  ( 0.000000000000000000, 0.000000000000000000, 1.000000000000000000 ) ) ;
#2236=VECTOR ( 'NONE', #9557, 1000.000000000000000 ) ;
#2240=ORIENTED_EDGE ( 'NONE', *, *, #3782, .F. ) ;
#2242=AXIS2_PLACEMENT_3D ( 'NONE', #12105, #11601, #8711 ) ;
#2245=DIRECTION ( 'NONE',  ( 0.000000000000000000, 0.000000000000000000, -1.000000000000000000 ) ) ;
#2246=VERTEX_POINT ( 'NONE', #10311 ) ;
#2247=FACE_OUTER_BOUND ( 'NONE', #12228, .T. ) ;
#2253=DIRECTION ( 'NONE',  ( -1.000000000000000000, -0.000000000000000000, -0.000000000000000000 ) ) ;
#2256=LINE ( 'NONE', #137, #5973 ) ;
#2258=CARTESIAN_POINT ( 'NONE',  ( 69.52686081653675387, 19.66584645497869843, 28.12499999996316546 ) ) ;
#2261=CARTESIAN_POINT ( 'NONE',  ( 69.53320273752093783, 40.66811906995093295, -28.10933780299387763 ) ) ;
#2265=PRODUCT_DEFINITION_CONTEXT ( 'detailed design', #5510, 'design' ) ;
#2267=CARTESIAN_POINT ( 'NONE',  ( 71.54748821555412519, 44.36552556075854881, 22.64388168110885857 ) ) ;
#2272=CARTESIAN_POINT ( 'NONE',  ( -23.51709844389219839, 11.48290155610792063, -57.08203932499370836 ) ) ;
#2280=EDGE_CURVE ( 'NONE', #2560, #5411, #8990, .T. ) ;
#2284=CIRCLE ( 'NONE', #697, 9.999999999999998224 ) ;
#2289=ORIENTED_EDGE ( 'NONE', *, *, #10112, .T. ) ;
#2299=ORIENTED_EDGE ( 'NONE', *, *, #3925, .T. ) ;
#2303=CARTESIAN_POINT ( 'NONE',  ( 70.07436679451828354, 45.25447089753193808, -26.73229126030999581 ) ) ;
#2306=ADVANCED_FACE ( 'NONE', ( #1220 ), #6079, .F. ) ;
#2308=ORIENTED_EDGE ( 'NONE', *, *, #6327, .T. ) ;
#2313=DIRECTION ( 'NONE',  ( 1.000000000000000000, 0.000000000000000000, 0.000000000000000000 ) ) ;
#2315=ORIENTED_EDGE ( 'NONE', *, *, #4354, .F. ) ;
#2317=CARTESIAN_POINT ( 'NONE',  ( 75.04559065614574820, 43.19565876339696331, -23.85935468423092587 ) ) ;
#2319=ORIENTED_EDGE ( 'NONE', *, *, #8930, .F. ) ;
#2321=CARTESIAN_POINT ( 'NONE',  ( 69.87020289360386016, 15.79423913611491948, 27.26117375607985593 ) ) ;
#2322=VECTOR ( 'NONE', #2139, 1000.000000000000000 ) ;
#2324=CARTESIAN_POINT ( 'NONE',  ( 76.84533340411822167, 44.87486296789415974, -21.12320159127844832 ) ) ;
#2328=CARTESIAN_POINT ( 'NONE',  ( 71.26470115309105324, 43.60909254972982296, 23.55923316143271151 ) ) ;
#2340=CARTESIAN_POINT ( 'NONE',  ( 30.00000000000004263, 65.00000000000000000, -57.08203932499370836 ) ) ;
#2345=CARTESIAN_POINT ( 'NONE',  ( 72.28493664348422953, 10.06798366438096615, -20.00732221823095003 ) ) ;
#2350=CIRCLE ( 'NONE', #6943, 70.00000000000001421 ) ;
#2354=VERTEX_POINT ( 'NONE', #5957 ) ;
#2356=CARTESIAN_POINT ( 'NONE',  ( 170.0000000000011369, 35.00000000000004974, 25.00000000000000000 ) ) ;
#2358=DIRECTION ( 'NONE',  ( 0.000000000000000000, -0.000000000000000000, 1.000000000000000000 ) ) ;
#2363=ADVANCED_FACE ( 'NONE', ( #1281 ), #9740, .F. ) ;
#2367=DIRECTION ( 'NONE',  ( 3.469446951953613203E-16, -0.000000000000000000, 1.000000000000000000 ) ) ;
#2371=LINE ( 'NONE', #8968, #9868 ) ;
#2373=LINE ( 'NONE', #8911, #7667 ) ;
#2378=CARTESIAN_POINT ( 'NONE',  ( 71.43334412524814070, 10.98941133951209892, 22.86096127246252863 ) ) ;
#2379=AXIS2_PLACEMENT_3D ( 'NONE', #1857, #4662, #7293 ) ;
#2380=ORIENTED_EDGE ( 'NONE', *, *, #7548, .T. ) ;
#2381=CARTESIAN_POINT ( 'NONE',  ( 71.78384618016781360, 49.48703820365247452, -21.72949947218331701 ) ) ;
#2385=CARTESIAN_POINT ( 'NONE',  ( 70.79098555896973721, 40.43144037915666900, 24.99999999902148318 ) ) ;
#2397=UNCERTAINTY_MEASURE_WITH_UNIT (LENGTH_MEASURE( 1.000000000000000082E-05 ), #218, 'distance_accuracy_value', 'NONE');
#2398=DIRECTION ( 'NONE',  ( 0.000000000000000000, 0.000000000000000000, -1.000000000000000000 ) ) ;
#2400=DIRECTION ( 'NONE',  ( 3.469446951953613203E-16, 0.000000000000000000, 1.000000000000000000 ) ) ;
#2407=CARTESIAN_POINT ( 'NONE',  ( 165.0000000000011369, 37.07106781186553945, 25.00000000000000000 ) ) ;
#2413=AXIS2_PLACEMENT_3D ( 'NONE', #8157, #7114, #1379 ) ;
#2417=DIRECTION ( 'NONE',  ( 0.000000000000000000, 1.000000000000000000, 0.000000000000000000 ) ) ;
#2421=ORIENTED_EDGE ( 'NONE', *, *, #6395, .T. ) ;
#2423=CARTESIAN_POINT ( 'NONE',  ( 170.0000000000011369, 230.0000000000000853, 20.00000000000000000 ) ) ;
#2426=EDGE_CURVE ( 'NONE', #9072, #8398, #11566, .T. ) ;
#2433=DIRECTION ( 'NONE',  ( -1.000000000000000000, -0.000000000000000000, 0.000000000000000000 ) ) ;
#2441=EDGE_CURVE ( 'NONE', #11288, #7839, #4685, .T. ) ;
#2442=( BOUNDED_CURVE ( )  B_SPLINE_CURVE ( 3, ( #2458, #9233, #10403, #4513 ),
 .UNSPECIFIED., .F., .F. ) 
 B_SPLINE_CURVE_WITH_KNOTS ( ( 4, 4 ),
 ( 1.570796326794899000, 3.141592653589793116 ),
 .UNSPECIFIED. ) 
 CURVE ( )  GEOMETRIC_REPRESENTATION_ITEM ( )  RATIONAL_B_SPLINE_CURVE ( ( 1.000000000000000000, 0.8047378541243654926, 0.8047378541243654926, 1.000000000000000000 ) ) 
 REPRESENTATION_ITEM ( '' )  );
#2449=CARTESIAN_POINT ( 'NONE',  ( 70.93011667421329491, 17.92389934224341630, 24.58871393576433206 ) ) ;
#2451=CARTESIAN_POINT ( 'NONE',  ( 75.70742691175847483, 15.93620156380750785, 22.92955197636053555 ) ) ;
#2455=CARTESIAN_POINT ( 'NONE',  ( 71.26309188267669015, 48.71650692501490454, 23.38502809576078079 ) ) ;
#2458=CARTESIAN_POINT ( 'NONE',  ( 147.9289321881356045, 20.00000000000008527, -25.00000000000000000 ) ) ;
#2465=ADVANCED_FACE ( 'NONE', ( #8298 ), #1802, .F. ) ;
#2468=DIRECTION ( 'NONE',  ( 0.000000000000000000, -1.000000000000000000, -0.000000000000000000 ) ) ;
#2471=CARTESIAN_POINT ( 'NONE',  ( 135.0000000000011084, 67.07106781186550393, -25.00000000000000000 ) ) ;
#2475=VECTOR ( 'NONE', #11753, 1000.000000000000000 ) ;
#2486=CARTESIAN_POINT ( 'NONE',  ( 74.16198487095667247, 19.63704101494498744, -25.00000000000000355 ) ) ;
#2493=AXIS2_PLACEMENT_3D ( 'NONE', #5634, #2634, #8539 ) ;
#2499=AXIS2_PLACEMENT_3D ( 'NONE', #10697, #1352, #10818 ) ;
#2500=ORIENTED_EDGE ( 'NONE', *, *, #10645, .T. ) ;
#2503=ORIENTED_EDGE ( 'NONE', *, *, #6785, .F. ) ;
#2505=LINE ( 'NONE', #8160, #4894 ) ;
#2510=CARTESIAN_POINT ( 'NONE',  ( 71.69575657208352482, 10.62176056569362537, 22.01828877003918450 ) ) ;
#2521=CARTESIAN_POINT ( 'NONE',  ( 71.99731494077012428, 45.04006870689263309, 21.09170898385188408 ) ) ;
#2528=ORIENTED_EDGE ( 'NONE', *, *, #11945, .F. ) ;
#2536=DIRECTION ( 'NONE',  ( 0.000000000000000000, 0.000000000000000000, 1.000000000000000000 ) ) ;
#2537=CARTESIAN_POINT ( 'NONE',  ( 69.89773400907222367, 15.60145727894099288, -27.19132888315842678 ) ) ;
#2540=EDGE_CURVE ( 'NONE', #12227, #834, #8356, .T. ) ;
#2542=CARTESIAN_POINT ( 'NONE',  ( 4.519788800730417222, 16.12168438296734152, 74.86496749433132436 ) ) ;
#2549=FACE_OUTER_BOUND ( 'NONE', #11279, .T. ) ;
#2555=LINE ( 'NONE', #5492, #8909 ) ;
#2556=CARTESIAN_POINT ( 'NONE',  ( -1.190781129305471087, 30.00000000000008882, 65.00000000000000000 ) ) ;
#2557=ORIENTED_EDGE ( 'NONE', *, *, #219, .F. ) ;
#2560=VERTEX_POINT ( 'NONE', #1945 ) ;
#2562=PLANE ( 'NONE',  #1081 ) ;
#2583=EDGE_CURVE ( 'NONE', #712, #5113, #4168, .T. ) ;
#2584=ORIENTED_EDGE ( 'NONE', *, *, #982, .T. ) ;
#2585=EDGE_CURVE ( 'NONE', #5113, #4639, #11142, .T. ) ;
#2588=DIRECTION ( 'NONE',  ( -0.000000000000000000, 1.000000000000000000, -0.000000000000000000 ) ) ;
#2594=CARTESIAN_POINT ( 'NONE',  ( 170.0000000000011369, 35.00000000000004974, -19.99999999999999645 ) ) ;
#2597=CARTESIAN_POINT ( 'NONE',  ( 69.62171139626217098, 17.74911263749020662, -27.88944765769274525 ) ) ;
#2603=AXIS2_PLACEMENT_3D ( 'NONE', #1344, #276, #6830 ) ;
#2605=CARTESIAN_POINT ( 'NONE',  ( 0.000000000000000000, 50.00000000000000000, 0.000000000000000000 ) ) ;
#2612=VECTOR ( 'NONE', #9033, 1000.000000000000000 ) ;
#2613=ORIENTED_EDGE ( 'NONE', *, *, #7746, .F. ) ;
#2618=ORIENTED_EDGE ( 'NONE', *, *, #405, .F. ) ;
#2623=EDGE_CURVE ( 'NONE', #1747, #10667, #1589, .T. ) ;
#2628=ORIENTED_EDGE ( 'NONE', *, *, #8128, .T. ) ;
#2634=DIRECTION ( 'NONE',  ( 0.000000000000000000, -1.000000000000000000, 0.000000000000000000 ) ) ;
#2637=CARTESIAN_POINT ( 'NONE',  ( 72.04420248082804790, 49.75119935390800663, 20.85013644286522094 ) ) ;
#2653=FACE_BOUND ( 'NONE', #1467, .T. ) ;
#2660=ORIENTED_EDGE ( 'NONE', *, *, #8890, .F. ) ;
#2665=CARTESIAN_POINT ( 'NONE',  ( 70.93313137955964010, 17.93151681614107318, -24.57887570927868026 ) ) ;
#2675=LINE ( 'NONE', #8339, #9004 ) ;
#2676=ORIENTED_EDGE ( 'NONE', *, *, #5111, .T. ) ;
#2682=DIRECTION ( 'NONE',  ( -1.000000000000000000, 0.000000000000000000, -3.469446951953613203E-16 ) ) ;
#2686=ORIENTED_EDGE ( 'NONE', *, *, #7352, .T. ) ;
#2695=CARTESIAN_POINT ( 'NONE',  ( 69.62171139626212835, 42.25088736250997101, 27.88944765769274170 ) ) ;
#2698=CARTESIAN_POINT ( 'NONE',  ( -20.00000000000004263, 54.99999999999999289, 67.08203932499370126 ) ) ;
#2701=DIRECTION ( 'NONE',  ( -0.7071067811865464625, 0.7071067811865486830, 2.453269466693394184E-16 ) ) ;
#2706=ORIENTED_EDGE ( 'NONE', *, *, #7986, .F. ) ;
#2709=LINE ( 'NONE', #7571, #6453 ) ;
#2710=LINE ( 'NONE', #3706, #8120 ) ;
#2721=EDGE_CURVE ( 'NONE', #7739, #5487, #9535, .T. ) ;
#2722=CARTESIAN_POINT ( 'NONE',  ( 3.645076725190190992, 15.79321527920849633, 74.91265089688103274 ) ) ;
#2727=CARTESIAN_POINT ( 'NONE',  ( 69.73318542092266625, 16.71298883719501305, -27.60965287711918492 ) ) ;
#2728=ORIENTED_EDGE ( 'NONE', *, *, #2745, .F. ) ;
#2731=ORIENTED_EDGE ( 'NONE', *, *, #937, .T. ) ;
#2733=CARTESIAN_POINT ( 'NONE',  ( 145.0000000000011369, 225.0000000000000853, -20.00000000000000000 ) ) ;
#2735=ORIENTED_EDGE ( 'NONE', *, *, #1498, .T. ) ;
#2736=DIRECTION ( 'NONE',  ( 0.000000000000000000, 0.5150380749100502698, 0.8571673007021147761 ) ) ;
#2737=FACE_OUTER_BOUND ( 'NONE', #6486, .T. ) ;
#2741=DIRECTION ( 'NONE',  ( -3.469446951953613203E-16, 0.000000000000000000, 1.000000000000000000 ) ) ;
#2743=SPHERICAL_SURFACE ( 'NONE', #4803, 5.000000000000000000 ) ;
#2744=CIRCLE ( 'NONE', #7733, 10.00000000000000888 ) ;
#2745=EDGE_CURVE ( 'NONE', #6757, #1244, #4738, .T. ) ;
#2749=CARTESIAN_POINT ( 'NONE',  ( 4.163799117101000559E-16, 115.0000000000000000, -3.399999999999999911 ) ) ;
#2753=CARTESIAN_POINT ( 'NONE',  ( -15.76450185945197902, 26.41238025498855180, 73.32456738963179532 ) ) ;
#2760=LINE ( 'NONE', #6387, #8487 ) ;
#2763=CARTESIAN_POINT ( 'NONE',  ( -20.00000000000000355, 50.00000000000000000, -57.08203932499370836 ) ) ;
#2768=VERTEX_POINT ( 'NONE', #5066 ) ;
#2780=CARTESIAN_POINT ( 'NONE',  ( 76.47547367680522257, 44.68911971724172361, -21.74308734404387167 ) ) ;
#2782=ORIENTED_EDGE ( 'NONE', *, *, #8591, .F. ) ;
#2785=DIRECTION ( 'NONE',  ( -1.000000000000000000, 0.000000000000000000, 0.000000000000000000 ) ) ;
#2788=AXIS2_PLACEMENT_3D ( 'NONE', #1329, #6997, #3952 ) ;
#2791=EDGE_CURVE ( 'NONE', #11350, #11684, #2744, .T. ) ;
#2793=ORIENTED_EDGE ( 'NONE', *, *, #5485, .T. ) ;
#2798=ORIENTED_EDGE ( 'NONE', *, *, #5540, .F. ) ;
#2799=CARTESIAN_POINT ( 'NONE',  ( 41.03553390593252459, -41.03553390593295802, 25.00000000000000000 ) ) ;
#2801=ORIENTED_EDGE ( 'NONE', *, *, #10352, .F. ) ;
#2805=ADVANCED_FACE ( 'NONE', ( #7970 ), #5245, .T. ) ;
#2810=CARTESIAN_POINT ( 'NONE',  ( 165.0000000000011369, 225.0000000000000853, -20.00000000000000000 ) ) ;
#2817=ADVANCED_FACE ( 'NONE', ( #436 ), #8031, .F. ) ;
#2820=CARTESIAN_POINT ( 'NONE',  ( 71.66575360104040726, 49.33907185937723483, 22.11578253505649982 ) ) ;
#2821=ORIENTED_EDGE ( 'NONE', *, *, #12269, .T. ) ;
#2836=ORIENTED_EDGE ( 'NONE', *, *, #2426, .T. ) ;
#2839=CARTESIAN_POINT ( 'NONE',  ( 1.836970198721029589E-15, 75.00000000000000000, 15.00000000000000000 ) ) ;
#2843=EDGE_CURVE ( 'NONE', #3680, #4047, #8403, .T. ) ;
#2845=CIRCLE ( 'NONE', #1461, 5.000000000000001776 ) ;
#2847=CARTESIAN_POINT ( 'NONE',  ( 71.30804307394106445, 43.76264759282432237, -23.42323195207071507 ) ) ;
#2859=EDGE_LOOP ( 'NONE', ( #11635, #11057, #12176, #7298 ) ) ;
#2873=AXIS2_PLACEMENT_3D ( 'NONE', #8702, #10456, #9697 ) ;
#2882=CARTESIAN_POINT ( 'NONE',  ( 69.71747094087791652, 16.79237370886442804, 27.65023488237563498 ) ) ;
#2884=LINE ( 'NONE', #2015, #10279 ) ;
#2886=DIRECTION ( 'NONE',  ( 0.000000000000000000, 0.000000000000000000, -1.000000000000000000 ) ) ;
#2892=EDGE_CURVE ( 'NONE', #8933, #8398, #3945, .T. ) ;
#2894=AXIS2_PLACEMENT_3D ( 'NONE', #2176, #117, #4992 ) ;
#2895=ORIENTED_EDGE ( 'NONE', *, *, #9499, .T. ) ;
#2896=STYLED_ITEM ( 'NONE', ( #10572 ), #482 ) ;
#2898=CARTESIAN_POINT ( 'NONE',  ( 3.197275507839122177, 44.35135159419116491, 74.93316431128972965 ) ) ;
#2906=EDGE_CURVE ( 'NONE', #10814, #5994, #9098, .T. ) ;
#2908=B_SPLINE_CURVE_WITH_KNOTS ( 'NONE', 3,
 ( #9291, #12303, #9411, #4565, #3, #11426, #2820, #11180, #1763, #1824, #12122, #3571, #7500, #6622, #1706, #12185, #892, #7618, #11246, #9350, #4750, #10417, #2695, #3818, #6507, #1880 ),
 .UNSPECIFIED., .F., .F.,
 ( 4, 2, 2, 2, 2, 2, 2, 2, 2, 2, 2, 2, 4 ),
 ( 1.040834085586084257E-17, 0.001946127227419483172, 0.002919190841129219553, 0.003892254454838955935, 0.005838381682258432168, 0.006811445295968166815, 0.007784508909677901461, 0.008757572523387635241, 0.009730636137097370755, 0.01167676336451683311, 0.01264982697822655995, 0.01362289059193628506, 0.01556901781935573353 ),
 .UNSPECIFIED. ) ;
#2909=CARTESIAN_POINT ( 'NONE',  ( 70.92179708824016870, 47.98984913414685849, -24.39594572817711438 ) ) ;
#2921=CARTESIAN_POINT ( 'NONE',  ( 8.572527594031474570E-15, 5.000000000000129674, -70.00000000000001421 ) ) ;
#2928=CARTESIAN_POINT ( 'NONE',  ( 74.16198487095664404, 40.36295898505520086, 25.00000000000000355 ) ) ;
#2929=EDGE_LOOP ( 'NONE', ( #328, #7017, #787 ) ) ;
#2935=PRODUCT_CONTEXT ( 'NONE', #10591, 'mechanical' ) ;
#2936=CARTESIAN_POINT ( 'NONE',  ( 145.0000000000011369, 225.0000000000000853, -25.00000000000000000 ) ) ;
#2944=CARTESIAN_POINT ( 'NONE',  ( 150.0000000000010800, 15.00000000000008882, -19.99999999999999645 ) ) ;
#2945=EDGE_LOOP ( 'NONE', ( #8906, #6831, #3725, #818 ) ) ;
#2946=CYLINDRICAL_SURFACE ( 'NONE', #831, 5.000000000000000888 ) ;
#2947=DIRECTION ( 'NONE',  ( -3.469446951953613696E-16, 0.000000000000000000, 1.000000000000000000 ) ) ;
#2952=EDGE_CURVE ( 'NONE', #9665, #9381, #2555, .T. ) ;
#2955=EDGE_CURVE ( 'NONE', #8153, #2768, #8281, .T. ) ;
#2960=DIRECTION ( 'NONE',  ( 0.000000000000000000, 0.000000000000000000, -1.000000000000000000 ) ) ;
#2961=CARTESIAN_POINT ( 'NONE',  ( 13.72352623184575293, 31.85795502388325673, 73.73395739868169585 ) ) ;
#2969=SURFACE_STYLE_FILL_AREA ( #9685 ) ;
#2971=ORIENTED_EDGE ( 'NONE', *, *, #5540, .T. ) ;
#2972=CARTESIAN_POINT ( 'NONE',  ( 70.44139041661959766, 46.67990480737745429, -25.75312943552223288 ) ) ;
#2977=LINE ( 'NONE', #10576, #8961 ) ;
#2978=CARTESIAN_POINT ( 'NONE',  ( 77.45966692414835109, 15.00000000000009059, -19.99999999999999645 ) ) ;
#2989=CARTESIAN_POINT ( 'NONE',  ( 75.52936542331360670, 43.86594787320247235, 23.18670291617644352 ) ) ;
#2990=EDGE_LOOP ( 'NONE', ( #1104, #11477 ) ) ;
#3003=DIRECTION ( 'NONE',  ( -0.000000000000000000, 1.000000000000000000, -0.000000000000000000 ) ) ;
#3008=DIRECTION ( 'NONE',  ( -0.9682458365518543664, 0.000000000000000000, -0.2499999999999996947 ) ) ;
#3021=DIRECTION ( 'NONE',  ( 0.000000000000000000, -1.000000000000000000, -0.000000000000000000 ) ) ;
#3027=CIRCLE ( 'NONE', #4215, 4.999999999999998224 ) ;
#3029=PLANE ( 'NONE',  #10359 ) ;
#3038=CARTESIAN_POINT ( 'NONE',  ( 75.38891993288051196, 16.31599220047735344, -23.38442328187116104 ) ) ;
#3044=CARTESIAN_POINT ( 'NONE',  ( 0.000000000000000000, 109.0000000000000000, 0.000000000000000000 ) ) ;
#3053=DIRECTION ( 'NONE',  ( 0.000000000000000000, 0.000000000000000000, -1.000000000000000000 ) ) ;
#3054=ORIENTED_EDGE ( 'NONE', *, *, #4953, .F. ) ;
#3060=CARTESIAN_POINT ( 'NONE',  ( 149.1421356237320026, 17.07106781186555722, 24.99999999999999645 ) ) ;
#3064=DIRECTION ( 'NONE',  ( 0.000000000000000000, 0.000000000000000000, -1.000000000000000000 ) ) ;
#3071=DIRECTION ( 'NONE',  ( -0.000000000000000000, -1.000000000000000000, -0.000000000000000000 ) ) ;
#3089=TOROIDAL_SURFACE ( 'NONE', #9039, 10.00000000000000000, 5.000000000000000000 ) ;
#3096=ORIENTED_EDGE ( 'NONE', *, *, #4197, .F. ) ;
#3100=CYLINDRICAL_SURFACE ( 'NONE', #9425, 15.00000000000000000 ) ;
#3102=CARTESIAN_POINT ( 'NONE',  ( 0.000000000000000000, 65.00000000000000000, 0.000000000000000000 ) ) ;
#3112=ORIENTED_EDGE ( 'NONE', *, *, #3965, .T. ) ;
#3119=EDGE_CURVE ( 'NONE', #11350, #8283, #876, .T. ) ;
#3128=FACE_OUTER_BOUND ( 'NONE', #7169, .T. ) ;
#3137=CARTESIAN_POINT ( 'NONE',  ( 3.517098443892134441, 31.48290155610792596, 57.08203932499370836 ) ) ;
#3139=EDGE_LOOP ( 'NONE', ( #10165, #8832, #1684, #4816 ) ) ;
#3145=ORIENTED_EDGE ( 'NONE', *, *, #6573, .F. ) ;
#3147=CARTESIAN_POINT ( 'NONE',  ( 0.000000000000000000, 0.000000000000000000, 25.00000000000000000 ) ) ;
#3149=LINE ( 'NONE', #2272, #12173 ) ;
#3159=CARTESIAN_POINT ( 'NONE',  ( 70.75727862648629696, 12.41690240222903618, -24.86906317558853274 ) ) ;
#3160=FACE_OUTER_BOUND ( 'NONE', #10147, .T. ) ;
#3173=CIRCLE ( 'NONE', #5775, 15.00000000000000000 ) ;
#3182=ORIENTED_EDGE ( 'NONE', *, *, #11643, .F. ) ;
#3187=DIRECTION ( 'NONE',  ( 0.000000000000000000, 0.000000000000000000, 1.000000000000000000 ) ) ;
#3189=CIRCLE ( 'NONE', #5978, 5.000000000000000888 ) ;
#3191=LINE ( 'NONE', #9029, #12268 ) ;
#3194=CARTESIAN_POINT ( 'NONE',  ( 76.05876219242703939, 44.39552472664445304, -22.40335076292606331 ) ) ;
#3199=CARTESIAN_POINT ( 'NONE',  ( 76.56943592554333122, 15.25648089810431429, 21.58906638518815768 ) ) ;
#3203=CARTESIAN_POINT ( 'NONE',  ( 75.04559065614574820, 16.80434123660322143, 23.85935468423092587 ) ) ;
#3204=CARTESIAN_POINT ( 'NONE',  ( 72.13972991039015881, 45.12505515914934051, -20.57104709750046467 ) ) ;
#3207=CARTESIAN_POINT ( 'NONE',  ( 70.52159520668648440, 46.91448669815612504, 25.52954545350316451 ) ) ;
#3217=AXIS2_PLACEMENT_3D ( 'NONE', #11462, #6429, #12168 ) ;
#3218=( BOUNDED_SURFACE ( )  B_SPLINE_SURFACE ( 3, 2, ( 
 ( #5544, #9322, #805 ),
 ( #4598, #3667, #7349 ),
 ( #3786, #12276, #5667 ),
 ( #930, #7413, #7529 ),
 ( #8270, #11337, #6416 ),
 ( #2727, #2665, #8513 ),
 ( #7588, #9446, #11149 ),
 ( #4720, #11399, #9263 ),
 ( #9507, #11589, #5040 ),
 ( #1978, #3974, #8818 ),
 ( #10638, #10578, #6907 ),
 ( #3917, #4917, #8700 ),
 ( #2107, #3850, #1173 ),
 ( #11707, #6777, #3038 ),
 ( #3159, #6842, #7713 ),
 ( #7771, #5729, #988 ),
 ( #229, #7651, #5788 ),
 ( #1233, #4849, #11525 ),
 ( #1111, #8636, #10453 ),
 ( #4038, #11464, #4974 ),
 ( #4782, #2165, #164 ),
 ( #5910, #8573, #10698 ),
 ( #287, #9695, #9572 ),
 ( #8759, #4096, #7831 ),
 ( #11649, #7888, #36 ),
 ( #2043, #5968, #2978 ) ),
 .UNSPECIFIED., .F., .F., .F. ) 
 B_SPLINE_SURFACE_WITH_KNOTS ( ( 4, 2, 2, 2, 2, 2, 2, 2, 2, 2, 2, 2, 4 ),
 ( 3, 3 ),
 ( 0.006382978049045519471, 0.008387885753076820827, 0.009390339605092470204, 0.01039279345710812132, 0.01239770116113942180, 0.01340015501315507118, 0.01440260886517072229, 0.01540506271718637341, 0.01640751656920202278, 0.01841242427323332501, 0.01941487812524897438, 0.02041733197726462723, 0.02242223968129592598 ),
 ( 0.000000000000000000, 1.000000000000000000 ),
 .UNSPECIFIED. ) 
 GEOMETRIC_REPRESENTATION_ITEM ( )  RATIONAL_B_SPLINE_SURFACE ( (
 ( 1.000000000000000000, 0.8291561975888499525, 1.000000000000000000),
 ( 1.000000000000000000, 0.8291533992853002966, 1.000000000000000000),
 ( 1.000000000000000000, 0.8281244206747362391, 1.000000000000000000),
 ( 1.000000000000000000, 0.8251351734919084580, 1.000000000000000000),
 ( 1.000000000000000000, 0.8238971056969858209, 1.000000000000000000),
 ( 1.000000000000000000, 0.8209398665854176214, 1.000000000000000000),
 ( 1.000000000000000000, 0.8192278287709251483, 1.000000000000000000),
 ( 1.000000000000000000, 0.8135208904818415077, 1.000000000000000000),
 ( 1.000000000000000000, 0.8089311958809365377, 1.000000000000000000),
 ( 1.000000000000000000, 0.8010155071010215400, 1.000000000000000000),
 ( 1.000000000000000000, 0.7981992791123722064, 1.000000000000000000),
 ( 1.000000000000000000, 0.7923673440970026016, 1.000000000000000000),
 ( 1.000000000000000000, 0.7893380284540298941, 1.000000000000000000),
 ( 1.000000000000000000, 0.7830853791993543922, 1.000000000000000000),
 ( 1.000000000000000000, 0.7798619748040643840, 1.000000000000000000),
 ( 1.000000000000000000, 0.7732488416061723546, 1.000000000000000000),
 ( 1.000000000000000000, 0.7698413672832561394, 1.000000000000000000),
 ( 1.000000000000000000, 0.7595660318243934173, 1.000000000000000000),
 ( 1.000000000000000000, 0.7526475626047379741, 1.000000000000000000),
 ( 1.000000000000000000, 0.7423381171275357238, 1.000000000000000000),
 ( 1.000000000000000000, 0.7389127554685743782, 1.000000000000000000),
 ( 1.000000000000000000, 0.7321112719850653150, 1.000000000000000000),
 ( 1.000000000000000000, 0.7287565628962849873, 1.000000000000000000),
 ( 1.000000000000000000, 0.7189979416186721428, 1.000000000000000000),
 ( 1.000000000000000000, 0.7128432726192915903, 1.000000000000000000),
 ( 1.000000000000000000, 0.7071067811865474617, 1.000000000000000000) ) ) 
 REPRESENTATION_ITEM ( '' )  SURFACE ( )  );
#3223=DIRECTION ( 'NONE',  ( 1.000000000000000000, -0.000000000000000000, 0.000000000000000000 ) ) ;
#3229=VERTEX_POINT ( 'NONE', #5219 ) ;
#3234=CARTESIAN_POINT ( 'NONE',  ( 75.19960992036260450, 16.56778241586094680, -23.64972750892604125 ) ) ;
#3236=CIRCLE ( 'NONE', #6618, 5.000000000000007105 ) ;
#3240=CARTESIAN_POINT ( 'NONE',  ( 69.71747094087790231, 43.20762629113575315, -27.65023488237562788 ) ) ;
#3242=DIRECTION ( 'NONE',  ( 0.000000000000000000, 0.000000000000000000, 1.000000000000000000 ) ) ;
#3243=DIRECTION ( 'NONE',  ( 0.000000000000000000, 0.000000000000000000, 1.000000000000000000 ) ) ;
#3246=CARTESIAN_POINT ( 'NONE',  ( 71.93667174376723494, 10.34708426542594140, 21.21818801319905745 ) ) ;
#3247=ORIENTED_EDGE ( 'NONE', *, *, #11041, .T. ) ;
#3248=CARTESIAN_POINT ( 'NONE',  ( 0.000000000000000000, -5.000000000000000000, 70.00000000000001421 ) ) ;
#3250=CARTESIAN_POINT ( 'NONE',  ( 140.0000000000011369, 30.00000000000008882, 25.00000000000000000 ) ) ;
#3252=ORIENTED_EDGE ( 'NONE', *, *, #7895, .F. ) ;
#3255=CARTESIAN_POINT ( 'NONE',  ( 75.38685631124154440, 16.31864566613397471, 23.38733102174731471 ) ) ;
#3257=CARTESIAN_POINT ( 'NONE',  ( 72.45695464226038496, 45.13428099848909625, -19.37542581275873843 ) ) ;
#3262=CARTESIAN_POINT ( 'NONE',  ( 69.73318542092245309, 43.28701116280399219, 27.60965287711969651 ) ) ;
#3276=CARTESIAN_POINT ( 'NONE',  ( 135.0000000000011084, 67.07106781186550393, 20.00000000000000000 ) ) ;
#3277=DIRECTION ( 'NONE',  ( 1.000000000000000000, 0.000000000000000000, 0.000000000000000000 ) ) ;
#3279=CARTESIAN_POINT ( 'NONE',  ( 26.76795759904968364, 61.76795759904965877, -64.77864552555394084 ) ) ;
#3280=AXIS2_PLACEMENT_3D ( 'NONE', #2008, #5815, #2245 ) ;
#3284=EDGE_CURVE ( 'NONE', #11288, #11474, #566, .T. ) ;
#3285=EDGE_CURVE ( 'NONE', #7839, #8096, #7998, .T. ) ;
#3296=DIRECTION ( 'NONE',  ( 0.000000000000000000, 0.000000000000000000, 1.000000000000000000 ) ) ;
#3298=ORIENTED_EDGE ( 'NONE', *, *, #2280, .F. ) ;
#3299=AXIS2_PLACEMENT_3D ( 'NONE', #9721, #257, #131 ) ;
#3301=CARTESIAN_POINT ( 'NONE',  ( 145.0000000000011369, 225.0000000000000853, 20.00000000000000000 ) ) ;
#3306=AXIS2_PLACEMENT_3D ( 'NONE', #6146, #4031, #11768 ) ;
#3307=ORIENTED_EDGE ( 'NONE', *, *, #6439, .F. ) ;
#3310=CARTESIAN_POINT ( 'NONE',  ( 0.000000000000000000, 10.00000000000017586, 0.000000000000000000 ) ) ;
#3322=CARTESIAN_POINT ( 'NONE',  ( 76.19556706709904859, 15.49470566993306520, 22.19251267860115462 ) ) ;
#3324=ORIENTED_EDGE ( 'NONE', *, *, #609, .T. ) ;
#3325=CARTESIAN_POINT ( 'NONE',  ( 72.53968727264539496, 45.08133313514087348, -19.05499925486959256 ) ) ;
#3329=CARTESIAN_POINT ( 'NONE',  ( 69.91894869711104832, 44.51764890176950473, 27.13685080543958250 ) ) ;
#3330=ORIENTED_EDGE ( 'NONE', *, *, #6412, .F. ) ;
#3331=EDGE_CURVE ( 'NONE', #7839, #934, #2710, .T. ) ;
#3338=ORIENTED_EDGE ( 'NONE', *, *, #7548, .F. ) ;
#3340=VERTEX_POINT ( 'NONE', #10308 ) ;
#3343=ADVANCED_FACE ( 'NONE', ( #4524 ), #11327, .F. ) ;
#3345=LINE ( 'NONE', #2340, #4651 ) ;
#3346=CARTESIAN_POINT ( 'NONE',  ( 20.00000000000000000, 54.99999999999999289, -67.08203932499371547 ) ) ;
#3348=DIRECTION ( 'NONE',  ( 2.213536252433181072E-16, 0.000000000000000000, 1.000000000000000000 ) ) ;
#3351=CARTESIAN_POINT ( 'NONE',  ( 72.45461974811382788, 10.00000000000009592, -19.38446435976419835 ) ) ;
#3361=LINE ( 'NONE', #7156, #7825 ) ;
#3369=CARTESIAN_POINT ( 'NONE',  ( 69.64721689463591758, 42.58935033937477499, -27.82591776719579357 ) ) ;
#3376=DIRECTION ( 'NONE',  ( -3.469446951953613203E-16, 0.000000000000000000, -1.000000000000000000 ) ) ;
#3379=DIRECTION ( 'NONE',  ( -0.7071067811865433539, 0.7071067811865517916, 0.000000000000000000 ) ) ;
#3384=EDGE_CURVE ( 'NONE', #5113, #712, #2350, .T. ) ;
#3385=CARTESIAN_POINT ( 'NONE',  ( 70.75630133281157441, 12.41939062735542976, 24.87185742758358487 ) ) ;
#3388=VERTEX_POINT ( 'NONE', #1901 ) ;
#3391=ORIENTED_EDGE ( 'NONE', *, *, #9205, .F. ) ;
#3392=LINE ( 'NONE', #9167, #5868 ) ;
#3393=CARTESIAN_POINT ( 'NONE',  ( 75.47443053502085775, 43.79154879885060581, 23.26350036030316559 ) ) ;
#3397=DIRECTION ( 'NONE',  ( 1.000000000000000000, -0.000000000000000000, 1.224646799147353207E-16 ) ) ;
#3411=AXIS2_PLACEMENT_3D ( 'NONE', #1384, #12050, #1573 ) ;
#3415=CARTESIAN_POINT ( 'NONE',  ( 70.19857488179017935, 14.21697453379132803, -26.40439979598029652 ) ) ;
#3421=AXIS2_PLACEMENT_3D ( 'NONE', #9941, #7277, #2536 ) ;
#3424=ORIENTED_EDGE ( 'NONE', *, *, #5151, .T. ) ;
#3427=VERTEX_POINT ( 'NONE', #7455 ) ;
#3431=DIRECTION ( 'NONE',  ( 1.000000000000000000, -0.000000000000000000, 0.000000000000000000 ) ) ;
#3435=CARTESIAN_POINT ( 'NONE',  ( 71.75867793008814033, 49.45719000729793891, -21.81257403104604720 ) ) ;
#3437=VECTOR ( 'NONE', #4645, 1000.000000000000000 ) ;
#3443=CARTESIAN_POINT ( 'NONE',  ( 71.40042903152234999, 11.04265768716983054, 22.96380533506443555 ) ) ;
#3444=ORIENTED_EDGE ( 'NONE', *, *, #7986, .T. ) ;
#3449=CARTESIAN_POINT ( 'NONE',  ( 74.70719529697694838, 17.45645769019468574, 24.30790125104220678 ) ) ;
#3455=CARTESIAN_POINT ( 'NONE',  ( 74.18968745904427919, 40.67159320117693966, 24.96588476870680751 ) ) ;
#3458=CARTESIAN_POINT ( 'NONE',  ( 8.572527594031472993E-15, 65.00000000000000000, -70.00000000000000000 ) ) ;
#3464=AXIS2_PLACEMENT_3D ( 'NONE', #8997, #7085, #3277 ) ;
#3467=CARTESIAN_POINT ( 'NONE',  ( 167.9289321881357182, 35.85786437626914847, -25.00000000000001066 ) ) ;
#3471=CARTESIAN_POINT ( 'NONE',  ( -12.12726286035689327, 40.31710753316119877, 74.01694684401550717 ) ) ;
#3472=CARTESIAN_POINT ( 'NONE',  ( 9.183067057334849181, 19.15551980836006152, 74.43651270773197837 ) ) ;
#3473=CARTESIAN_POINT ( 'NONE',  ( 69.65097664248530407, 17.43447699930461425, -27.81636932325740474 ) ) ;
#3478=AXIS2_PLACEMENT_3D ( 'NONE', #10231, #5695, #8419 ) ;
#3483=CARTESIAN_POINT ( 'NONE',  ( 75.52936542331363512, 16.13405212679771239, -23.18670291617644708 ) ) ;
#3487=EDGE_CURVE ( 'NONE', #9722, #5183, #10575, .T. ) ;
#3502=AXIS2_PLACEMENT_3D ( 'NONE', #845, #4638, #1893 ) ;
#3509=CARTESIAN_POINT ( 'NONE',  ( 74.16198487095664404, 20.00000000000009237, 25.00000000000000000 ) ) ;
#3511=B_SPLINE_CURVE_WITH_KNOTS ( 'NONE', 3,
 ( #8357, #8300, #7440, #10294, #4627, #2753, #12243, #3690, #11307, #6561, #11552, #2133, #6056, #1014, #10786, #7910, #4815, #4880, #8603, #7677, #3879, #64, #1198, #1140, #9783, #5876, #5001, #7803 ),
 .UNSPECIFIED., .F., .F.,
 ( 4, 2, 2, 2, 2, 2, 2, 2, 2, 2, 2, 2, 2, 4 ),
 ( 0.06933356886758795801, 0.07087674937109647577, 0.07241992987460497966, 0.07396311037811349742, 0.07550629088162201519, 0.07859265188863905072, 0.08013583239214755460, 0.08167901289565607237, 0.08476537390267309402, 0.08630855440618159791, 0.08785173490969010179, 0.08939491541319860568, 0.09093809591670712345, 0.09402445692372414510 ),
 .UNSPECIFIED. ) ;
#3519=DIRECTION ( 'NONE',  ( -0.000000000000000000, 1.000000000000000000, -0.000000000000000000 ) ) ;
#3522=CARTESIAN_POINT ( 'NONE',  ( 1.530808498934191127E-15, 115.0000000000000000, -9.999999999999998224 ) ) ;
#3531=LINE ( 'NONE', #790, #3437 ) ;
#3534=CARTESIAN_POINT ( 'NONE',  ( -4.117654238873405426, 44.72076144782612772, 74.88857929402055902 ) ) ;
#3536=CARTESIAN_POINT ( 'NONE',  ( 70.48329812536721306, 13.20517121183804043, -25.63505613512332815 ) ) ;
#3546=ORIENTED_EDGE ( 'NONE', *, *, #5485, .F. ) ;
#3547=CYLINDRICAL_SURFACE ( 'NONE', #1484, 4.999999999999997335 ) ;
#3548=FACE_OUTER_BOUND ( 'NONE', #3872, .T. ) ;
#3549=ORIENTED_EDGE ( 'NONE', *, *, #7403, .F. ) ;
#3552=VERTEX_POINT ( 'NONE', #10745 ) ;
#3560=EDGE_CURVE ( 'NONE', #3822, #6450, #5960, .T. ) ;
#3562=CARTESIAN_POINT ( 'NONE',  ( -20.00000000000000355, 63.00000000000000000, -57.08203932499370836 ) ) ;
#3571=CARTESIAN_POINT ( 'NONE',  ( 70.71657310242181893, 47.47535718540355987, 24.98455589012892375 ) ) ;
#3572=ORIENTED_EDGE ( 'NONE', *, *, #5190, .T. ) ;
#3575=VERTEX_POINT ( 'NONE', #1962 ) ;
#3582=EDGE_CURVE ( 'NONE', #4047, #1244, #9802, .T. ) ;
#3587=CARTESIAN_POINT ( 'NONE',  ( 117.9289321881355193, 50.00000000000008527, 25.00000000000000000 ) ) ;
#3588=ADVANCED_FACE ( 'NONE', ( #5327 ), #9193, .F. ) ;
#3599=AXIS2_PLACEMENT_3D ( 'NONE', #10549, #2253, #9668 ) ;
#3602=DIRECTION ( 'NONE',  ( 0.000000000000000000, 0.000000000000000000, 1.000000000000000000 ) ) ;
#3603=EDGE_CURVE ( 'NONE', #11761, #12227, #12248, .T. ) ;
#3604=DIRECTION ( 'NONE',  ( 0.000000000000000000, 0.000000000000000000, -1.000000000000000000 ) ) ;
#3606=CARTESIAN_POINT ( 'NONE',  ( 63.96446609406733330, -63.96446609406769568, -20.00000000000000000 ) ) ;
#3618=ORIENTED_EDGE ( 'NONE', *, *, #7585, .F. ) ;
#3624=CARTESIAN_POINT ( 'NONE',  ( 8.572527594031472993E-15, 63.00000000000000000, -70.00000000000000000 ) ) ;
#3630=EDGE_CURVE ( 'NONE', #834, #8527, #5778, .T. ) ;
#3634=CARTESIAN_POINT ( 'NONE',  ( 9.184850993605150311E-15, 10.00000000000017586, 75.00000000000001421 ) ) ;
#3636=ORIENTED_EDGE ( 'NONE', *, *, #8930, .T. ) ;
#3638=FACE_OUTER_BOUND ( 'NONE', #9661, .T. ) ;
#3658=B_SPLINE_CURVE_WITH_KNOTS ( 'NONE', 3,
 ( #5143, #4314, #10988, #2202, #6255, #8109, #8919, #2451, #7988, #11934, #3203, #9985, #7003, #10045, #6191, #451, #6012, #576 ),
 .UNSPECIFIED., .F., .F.,
 ( 4, 2, 2, 2, 2, 2, 2, 2, 4 ),
 ( 0.000000000000000000, 0.001070780962355597247, 0.002141561924711194494, 0.003212342887066791525, 0.004283123849422388989, 0.005353904811777986453, 0.006424685774133583049, 0.007495466736489180513, 0.008566247698844777977 ),
 .UNSPECIFIED. ) ;
#3660=EDGE_LOOP ( 'NONE', ( #1072, #12123, #3182, #9979 ) ) ;
#3661=EDGE_CURVE ( 'NONE', #9442, #10391, #1714, .T. ) ;
#3664=AXIS2_PLACEMENT_3D ( 'NONE', #3899, #11508, #2960 ) ;
#3666=DIRECTION ( 'NONE',  ( 0.000000000000000000, 1.000000000000000000, 0.000000000000000000 ) ) ;
#3667=CARTESIAN_POINT ( 'NONE',  ( 70.79098555896973721, 19.56855962084436129, -24.99999999902147962 ) ) ;
#3669=DIRECTION ( 'NONE',  ( 0.000000000000000000, 0.000000000000000000, -1.000000000000000000 ) ) ;
#3671=ORIENTED_EDGE ( 'NONE', *, *, #1063, .T. ) ;
#3672=CARTESIAN_POINT ( 'NONE',  ( 147.9289321881356045, 20.00000000000009237, 25.00000000000000000 ) ) ;
#3678=ORIENTED_EDGE ( 'NONE', *, *, #7495, .F. ) ;
#3680=VERTEX_POINT ( 'NONE', #10236 ) ;
#3686=FACE_OUTER_BOUND ( 'NONE', #10497, .T. ) ;
#3687=ADVANCED_FACE ( 'NONE', ( #8422, #896 ), #3693, .T. ) ;
#3690=CARTESIAN_POINT ( 'NONE',  ( -15.31872880306210583, 24.93376880718456334, 73.41908715900406435 ) ) ;
#3691=EDGE_LOOP ( 'NONE', ( #9508, #12132, #4184, #10714 ) ) ;
#3693=PLANE ( 'NONE',  #2112 ) ;
#3696=DIRECTION ( 'NONE',  ( 3.469446951953613203E-16, -0.000000000000000000, 1.000000000000000000 ) ) ;
#3702=TOROIDAL_SURFACE ( 'NONE', #10668, 10.00000000000000000, 5.000000000000000000 ) ;
#3706=CARTESIAN_POINT ( 'NONE',  ( 63.96446609406734751, -63.96446609406770989, -25.00000000000000000 ) ) ;
#3721=ORIENTED_EDGE ( 'NONE', *, *, #2123, .T. ) ;
#3725=ORIENTED_EDGE ( 'NONE', *, *, #11408, .F. ) ;
#3728=VERTEX_POINT ( 'NONE', #7681 ) ;
#3730=B_SPLINE_CURVE_WITH_KNOTS ( 'NONE', 3,
 ( #8145, #2486, #6350, #1428, #6227, #9894, #8022, #10898, #3234, #3483, #11968, #10137, #7100, #6290, #11022, #5234, #10078, #11849 ),
 .UNSPECIFIED., .F., .F.,
 ( 4, 2, 2, 2, 2, 2, 2, 2, 4 ),
 ( 0.000000000000000000, 0.001070893387785249720, 0.002141786775570499440, 0.003212680163355748943, 0.004283573551140998879, 0.005354466938926247949, 0.006425360326711500487, 0.007496253714496753026, 0.008567147102282004698 ),
 .UNSPECIFIED. ) ;
#3748=AXIS2_PLACEMENT_3D ( 'NONE', #11196, #849, #8434 ) ;
#3751=FACE_OUTER_BOUND ( 'NONE', #9923, .T. ) ;
#3756=EDGE_CURVE ( 'NONE', #10965, #10533, #5107, .T. ) ;
#3757=EDGE_CURVE ( 'NONE', #10391, #8715, #11496, .T. ) ;
#3763=ORIENTED_EDGE ( 'NONE', *, *, #8591, .T. ) ;
#3772=CARTESIAN_POINT ( 'NONE',  ( 0.000000000000000000, -10.00000000000000000, 0.000000000000000000 ) ) ;
#3778=CARTESIAN_POINT ( 'NONE',  ( 69.52686081652184669, 40.00000000000008527, -28.12500000000000000 ) ) ;
#3780=FILL_AREA_STYLE ('',( #10448 ) ) ;
#3782=EDGE_CURVE ( 'NONE', #4212, #10619, #512, .T. ) ;
#3786=CARTESIAN_POINT ( 'NONE',  ( 69.55283199277543815, 18.65681359763190628, -28.06103394134222029 ) ) ;
#3789=CARTESIAN_POINT ( 'NONE',  ( 135.0000000000011084, 67.07106781186550393, -19.99999999999999645 ) ) ;
#3790=PRODUCT_DEFINITION_SHAPE ( 'NONE', 'NONE',  #11834 ) ;
#3793=EDGE_LOOP ( 'NONE', ( #2895, #3636 ) ) ;
#3795=VECTOR ( 'NONE', #2078, 1000.000000000000000 ) ;
#3796=( GEOMETRIC_REPRESENTATION_CONTEXT ( 3 ) GLOBAL_UNCERTAINTY_ASSIGNED_CONTEXT ( ( #6268 ) ) GLOBAL_UNIT_ASSIGNED_CONTEXT ( ( #10444, #2155, #1910 ) ) REPRESENTATION_CONTEXT ( 'NONE', 'WORKASPACE' ) );
#3808=DIRECTION ( 'NONE',  ( 0.000000000000000000, 0.000000000000000000, -1.000000000000000000 ) ) ;
#3809=DIRECTION ( 'NONE',  ( -1.000000000000000000, 0.000000000000000000, -6.938893903907222461E-16 ) ) ;
#3815=CIRCLE ( 'NONE', #1228, 5.000000000000000888 ) ;
#3818=CARTESIAN_POINT ( 'NONE',  ( 69.55111042745878080, 41.29936696797726370, 28.06526308249823032 ) ) ;
#3822=VERTEX_POINT ( 'NONE', #1949 ) ;
#3828=CARTESIAN_POINT ( 'NONE',  ( 142.0710678118665555, 59.99999999999998579, 25.00000000000000000 ) ) ;
#3831=EDGE_CURVE ( 'NONE', #6555, #8595, #11016, .T. ) ;
#3832=ORIENTED_EDGE ( 'NONE', *, *, #6310, .T. ) ;
#3842=ORIENTED_EDGE ( 'NONE', *, *, #3284, .T. ) ;
#3846=DIRECTION ( 'NONE',  ( 0.000000000000000000, 0.000000000000000000, -1.000000000000000000 ) ) ;
#3849=LINE ( 'NONE', #6717, #2102 ) ;
#3850=CARTESIAN_POINT ( 'NONE',  ( 71.45054378765421177, 15.85863886173339665, -22.96278406504537628 ) ) ;
#3851=ORIENTED_EDGE ( 'NONE', *, *, #8061, .F. ) ;
#3863=ORIENTED_EDGE ( 'NONE', *, *, #9304, .F. ) ;
#3868=CARTESIAN_POINT ( 'NONE',  ( 0.000000000000000000, 115.0000000000000000, 0.000000000000000000 ) ) ;
#3872=EDGE_LOOP ( 'NONE', ( #3252, #8206, #4079, #10496 ) ) ;
#3877=EDGE_CURVE ( 'NONE', #1231, #8595, #7485, .T. ) ;
#3878=DIRECTION ( 'NONE',  ( -1.000000000000000000, 0.000000000000000000, 0.000000000000000000 ) ) ;
#3879=CARTESIAN_POINT ( 'NONE',  ( -6.601480288436279764, 16.00045772279125700, 74.71048470746850967 ) ) ;
#3880=AXIS2_PLACEMENT_3D ( 'NONE', #8204, #8144, #5420 ) ;
#3883=DIRECTION ( 'NONE',  ( 0.000000000000000000, 0.000000000000000000, -1.000000000000000000 ) ) ;
#3884=CARTESIAN_POINT ( 'NONE',  ( 69.52686081652184669, 20.00000000000009237, 28.12499999999999645 ) ) ;
#3887=EDGE_CURVE ( 'NONE', #3680, #4313, #2371, .T. ) ;
#3892=CARTESIAN_POINT ( 'NONE',  ( 72.45695464226038496, 14.86571900151108494, 19.37542581275875619 ) ) ;
#3893=AXIS2_PLACEMENT_3D ( 'NONE', #1145, #10609, #1782 ) ;
#3894=EDGE_LOOP ( 'NONE', ( #4612, #6603, #3763, #8179, #7992 ) ) ;
#3896=VECTOR ( 'NONE', #6432, 1000.000000000000000 ) ;
#3897=ADVANCED_FACE ( 'NONE', ( #8035 ), #317, .T. ) ;
#3899=CARTESIAN_POINT ( 'NONE',  ( 74.16198487095665826, 50.00000000000000000, 30.00000000000000355 ) ) ;
#3900=CARTESIAN_POINT ( 'NONE',  ( 12.41779361890942290, 36.32650217634261480, 73.96515157582260258 ) ) ;
#3909=ORIENTED_EDGE ( 'NONE', *, *, #2745, .T. ) ;
#3911=CARTESIAN_POINT ( 'NONE',  ( 69.55864520994430222, 41.33566892181104890, -28.04631938806055658 ) ) ;
#3917=CARTESIAN_POINT ( 'NONE',  ( 70.44624282194224918, 13.32395845803458734, -25.73656789697610137 ) ) ;
#3925=EDGE_CURVE ( 'NONE', #11877, #6026, #565, .T. ) ;
#3926=VERTEX_POINT ( 'NONE', #8158 ) ;
#3928=CARTESIAN_POINT ( 'NONE',  ( 75.19960992036259029, 43.43221758413923794, 23.64972750892604481 ) ) ;
#3934=LINE ( 'NONE', #5685, #11191 ) ;
#3939=ORIENTED_EDGE ( 'NONE', *, *, #3603, .T. ) ;
#3941=DIRECTION ( 'NONE',  ( 0.000000000000000000, 1.000000000000000000, 0.000000000000000000 ) ) ;
#3945=CIRCLE ( 'NONE', #4945, 9.999999999999998224 ) ;
#3947=EDGE_CURVE ( 'NONE', #7739, #44, #3191, .T. ) ;
#3952=DIRECTION ( 'NONE',  ( 0.000000000000000000, 0.000000000000000000, 1.000000000000000000 ) ) ;
#3958=DIRECTION ( 'NONE',  ( 0.000000000000000000, -0.000000000000000000, 1.000000000000000000 ) ) ;
#3960=ORIENTED_EDGE ( 'NONE', *, *, #8475, .T. ) ;
#3962=FACE_OUTER_BOUND ( 'NONE', #12167, .T. ) ;
#3965=EDGE_CURVE ( 'NONE', #3926, #11761, #8908, .T. ) ;
#3968=CARTESIAN_POINT ( 'NONE',  ( 74.58430552651930157, 42.25186411422790655, -24.46729545492062385 ) ) ;
#3974=CARTESIAN_POINT ( 'NONE',  ( 71.26470115309105324, 16.39090745027094798, -23.55923316143329416 ) ) ;
#3979=EDGE_LOOP ( 'NONE', ( #4172, #2289, #11702, #5545, #11579, #5316, #4614, #10830 ) ) ;
#3982=ORIENTED_EDGE ( 'NONE', *, *, #4713, .F. ) ;
#3986=LINE ( 'NONE', #6667, #250 ) ;
#3993=CARTESIAN_POINT ( 'NONE',  ( 117.9289321881355193, 40.00000000000009237, -25.00000000000000000 ) ) ;
#4000=DIRECTION ( 'NONE',  ( -1.224646799147354193E-16, 0.000000000000000000, -1.000000000000000000 ) ) ;
#4006=ORIENTED_EDGE ( 'NONE', *, *, #6267, .T. ) ;
#4010=CARTESIAN_POINT ( 'NONE',  ( 117.9289321881355193, 50.00000000000008527, -25.00000000000000000 ) ) ;
#4011=LINE ( 'NONE', #3137, #7949 ) ;
#4019=CARTESIAN_POINT ( 'NONE',  ( 10.45882351999534521, 39.49462622639263287, 74.26988840762503230 ) ) ;
#4020=VERTEX_POINT ( 'NONE', #8466 ) ;
#4028=DIRECTION ( 'NONE',  ( 0.000000000000000000, 1.000000000000000000, 0.000000000000000000 ) ) ;
#4031=DIRECTION ( 'NONE',  ( -0.000000000000000000, -1.000000000000000000, -0.000000000000000000 ) ) ;
#4035=ORIENTED_EDGE ( 'NONE', *, *, #9787, .F. ) ;
#4038=CARTESIAN_POINT ( 'NONE',  ( 71.69683552452198683, 10.62043640550095702, -22.01474836615561514 ) ) ;
#4039=ORIENTED_EDGE ( 'NONE', *, *, #6697, .T. ) ;
#4041=DIRECTION ( 'NONE',  ( 0.000000000000000000, 0.000000000000000000, -1.000000000000000000 ) ) ;
#4042=AXIS2_PLACEMENT_3D ( 'NONE', #9843, #8032, #1319 ) ;
#4043=ORIENTED_EDGE ( 'NONE', *, *, #1673, .F. ) ;
#4045=ADVANCED_FACE ( 'NONE', ( #11165 ), #1629, .F. ) ;
#4047=VERTEX_POINT ( 'NONE', #10336 ) ;
#4064=CARTESIAN_POINT ( 'NONE',  ( 170.0000000000011369, 35.00000000000004974, 20.00000000000000000 ) ) ;
#4079=ORIENTED_EDGE ( 'NONE', *, *, #8272, .F. ) ;
#4081=CARTESIAN_POINT ( 'NONE',  ( 11.99804506437387985, 37.16050278248236793, 74.03439849576338361 ) ) ;
#4085=CARTESIAN_POINT ( 'NONE',  ( 74.16198487095665826, 40.00000000000009237, -30.00000000000000355 ) ) ;
#4087=VECTOR ( 'NONE', #12233, 1000.000000000000000 ) ;
#4090=DIRECTION ( 'NONE',  ( 0.000000000000000000, 0.000000000000000000, -1.000000000000000000 ) ) ;
#4092=DIRECTION ( 'NONE',  ( -0.000000000000000000, 1.000000000000000000, -0.000000000000000000 ) ) ;
#4096=CARTESIAN_POINT ( 'NONE',  ( 72.45821416003295212, 14.86625829596107984, -19.37058730516337235 ) ) ;
#4109=CARTESIAN_POINT ( 'NONE',  ( 135.0000000000011084, 67.07106781186550393, 20.00000000000000000 ) ) ;
#4122=DIRECTION ( 'NONE',  ( 0.000000000000000000, 0.000000000000000000, 1.000000000000000000 ) ) ;
#4128=CARTESIAN_POINT ( 'NONE',  ( 76.59657895567488595, 44.76487798575835342, -21.54700147973310820 ) ) ;
#4132=CARTESIAN_POINT ( 'NONE',  ( 74.98307306353127899, 16.90879164695958892, 23.94359236838928240 ) ) ;
#4134=FACE_OUTER_BOUND ( 'NONE', #1861, .T. ) ;
#4136=EDGE_CURVE ( 'NONE', #3575, #7739, #10652, .T. ) ;
#4139=CARTESIAN_POINT ( 'NONE',  ( 69.55283199277504025, 41.34318640236479325, 28.06103394134322571 ) ) ;
#4140=ORIENTED_EDGE ( 'NONE', *, *, #3877, .F. ) ;
#4143=CARTESIAN_POINT ( 'NONE',  ( 0.000000000000000000, 109.0000000000000000, 0.000000000000000000 ) ) ;
#4144=CARTESIAN_POINT ( 'NONE',  ( 0.000000000000000000, 65.00000000000000000, 0.000000000000000000 ) ) ;
#4152=DIRECTION ( 'NONE',  ( -0.000000000000000000, 1.000000000000000000, -0.000000000000000000 ) ) ;
#4153=DIRECTION ( 'NONE',  ( 0.000000000000000000, 0.000000000000000000, 1.000000000000000000 ) ) ;
#4155=DIRECTION ( 'NONE',  ( 0.000000000000000000, 0.000000000000000000, 1.000000000000000000 ) ) ;
#4165=ORIENTED_EDGE ( 'NONE', *, *, #2791, .F. ) ;
#4167=AXIS2_PLACEMENT_3D ( 'NONE', #8149, #11971, #8898 ) ;
#4168=CIRCLE ( 'NONE', #11343, 70.00000000000001421 ) ;
#4172=ORIENTED_EDGE ( 'NONE', *, *, #4544, .F. ) ;
#4182=CARTESIAN_POINT ( 'NONE',  ( 117.9289321881355193, 50.00000000000008527, 25.00000000000000000 ) ) ;
#4183=CARTESIAN_POINT ( 'NONE',  ( 140.0000000000011369, 230.0000000000000853, 25.00000000000000000 ) ) ;
#4184=ORIENTED_EDGE ( 'NONE', *, *, #854, .T. ) ;
#4190=CARTESIAN_POINT ( 'NONE',  ( 0.000000000000000000, 110.0000000000000000, 0.000000000000000000 ) ) ;
#4191=AXIS2_PLACEMENT_3D ( 'NONE', #3772, #5777, #5715 ) ;
#4192=CARTESIAN_POINT ( 'NONE',  ( 74.16198487097054226, 19.83292322748416581, 25.00000000000000000 ) ) ;
#4197=EDGE_CURVE ( 'NONE', #6619, #3427, #4675, .T. ) ;
#4198=CARTESIAN_POINT ( 'NONE',  ( 75.38685631124155861, 43.68135433386650135, -23.38733102174701983 ) ) ;
#4201=CARTESIAN_POINT ( 'NONE',  ( 69.52686081652184669, 40.00000000000009237, 28.12500000000000000 ) ) ;
#4203=LINE ( 'NONE', #2149, #6222 ) ;
#4208=VECTOR ( 'NONE', #10220, 1000.000000000000000 ) ;
#4212=VERTEX_POINT ( 'NONE', #6226 ) ;
#4215=AXIS2_PLACEMENT_3D ( 'NONE', #10092, #4555, #9340 ) ;
#4216=CARTESIAN_POINT ( 'NONE',  ( 117.9289321881355193, 50.00000000000008527, 20.00000000000000000 ) ) ;
#4235=ADVANCED_FACE ( 'NONE', ( #7958 ), #3089, .T. ) ;
#4239=CARTESIAN_POINT ( 'NONE',  ( 69.52686081652184669, 20.00000000000009237, 28.12499999999999645 ) ) ;
#4245=LINE ( 'NONE', #10792, #2322 ) ;
#4250=CARTESIAN_POINT ( 'NONE',  ( 70.92179708824001239, 12.01015086585302960, 24.39594572817764373 ) ) ;
#4255=AXIS2_PLACEMENT_3D ( 'NONE', #9676, #4957, #3958 ) ;
#4260=CARTESIAN_POINT ( 'NONE',  ( 70.23094937779826807, 45.91093084162184823, 26.31821466697815382 ) ) ;
#4264=FACE_OUTER_BOUND ( 'NONE', #11353, .T. ) ;
#4269=ORIENTED_EDGE ( 'NONE', *, *, #3887, .T. ) ;
#4273=CARTESIAN_POINT ( 'NONE',  ( 117.9289321881355193, 50.00000000000008527, 20.00000000000000000 ) ) ;
#4281=CARTESIAN_POINT ( 'NONE',  ( 11.02471948819644965, 21.24513208498732908, 74.18696493688197791 ) ) ;
#4291=CARTESIAN_POINT ( 'NONE',  ( 120.0000000000009948, 45.00000000000008527, 25.00000000000000000 ) ) ;
#4293=DIRECTION ( 'NONE',  ( 0.000000000000000000, -1.000000000000000000, 0.000000000000000000 ) ) ;
#4301=DIRECTION ( 'NONE',  ( 0.7071067811865447972, -0.7071067811865503483, 0.000000000000000000 ) ) ;
#4311=CARTESIAN_POINT ( 'NONE',  ( 71.17928254424890611, 16.69380110197859324, 23.82724229592415810 ) ) ;
#4313=VERTEX_POINT ( 'NONE', #9829 ) ;
#4314=CARTESIAN_POINT ( 'NONE',  ( 77.29385721799278031, 15.00000000000008704, 20.32108911529004303 ) ) ;
#4318=CARTESIAN_POINT ( 'NONE',  ( 70.75727862648629696, 47.58309759777085901, 24.86906317558853630 ) ) ;
#4323=ADVANCED_FACE ( 'NONE', ( #1791 ), #10077, .T. ) ;
#4335=CARTESIAN_POINT ( 'NONE',  ( 74.16198487095665826, 40.00000000000009237, -25.00000000000000000 ) ) ;
#4348=ORIENTED_EDGE ( 'NONE', *, *, #7430, .T. ) ;
#4349=DIRECTION ( 'NONE',  ( 1.000000000000000000, 0.000000000000000000, 0.000000000000000000 ) ) ;
#4352=CARTESIAN_POINT ( 'NONE',  ( 72.61843774138907293, 50.00000000000000000, -18.75000000000000000 ) ) ;
#4354=EDGE_CURVE ( 'NONE', #5087, #5348, #294, .T. ) ;
#4356=DIRECTION ( 'NONE',  ( 1.000000000000000000, 0.000000000000000000, 0.000000000000000000 ) ) ;
#4360=AXIS2_PLACEMENT_3D ( 'NONE', #2471, #12139, #12202 ) ;
#4362=DIRECTION ( 'NONE',  ( 0.000000000000000000, 0.000000000000000000, 1.000000000000000000 ) ) ;
#4363=CARTESIAN_POINT ( 'NONE',  ( 166.4644660940684275, 38.53553390593280881, 25.00000000000000000 ) ) ;
#4367=CARTESIAN_POINT ( 'NONE',  ( 0.000000000000000000, 63.00000000000000000, -57.08203932499371547 ) ) ;
#4370=CARTESIAN_POINT ( 'NONE',  ( 76.84533340411822167, 15.12513703210600369, 21.12320159127833819 ) ) ;
#4378=CARTESIAN_POINT ( 'NONE',  ( 125.0000000000009663, 42.92893218813456713, -25.00000000000000000 ) ) ;
#4379=CARTESIAN_POINT ( 'NONE',  ( 75.22303488722339182, 43.45724334910113384, 23.61575757524099117 ) ) ;
#4399=CARTESIAN_POINT ( 'NONE',  ( 10.46236448685246856, 20.50957335928671199, 74.26939691374536778 ) ) ;
#4404=VECTOR ( 'NONE', #9001, 1000.000000000000114 ) ;
#4407=ORIENTED_EDGE ( 'NONE', *, *, #6024, .T. ) ;
#4414=CYLINDRICAL_SURFACE ( 'NONE', #11647, 5.000000000000004441 ) ;
#4420=EDGE_CURVE ( 'NONE', #8153, #6043, #12254, .T. ) ;
#4421=EDGE_LOOP ( 'NONE', ( #391, #9636, #6136, #5232 ) ) ;
#4422=VECTOR ( 'NONE', #8526, 1000.000000000000000 ) ;
#4428=VERTEX_POINT ( 'NONE', #11967 ) ;
#4442=CARTESIAN_POINT ( 'NONE',  ( -23.42809864819168553, 58.42809864819167132, 66.05997777686947359 ) ) ;
#4443=VECTOR ( 'NONE', #8068, 1000.000000000000000 ) ;
#4444=ORIENTED_EDGE ( 'NONE', *, *, #6773, .T. ) ;
#4465=AXIS2_PLACEMENT_3D ( 'NONE', #11776, #11837, #4155 ) ;
#4472=ORIENTED_EDGE ( 'NONE', *, *, #2892, .F. ) ;
#4478=CARTESIAN_POINT ( 'NONE',  ( 170.0000000000011369, 35.00000000000004974, 25.00000000000000000 ) ) ;
#4485=ORIENTED_EDGE ( 'NONE', *, *, #6327, .F. ) ;
#4496=CLOSED_SHELL ( 'NONE', ( #8874, #1856, #6733, #11048, #225, #5932, #1394, #5933, #2805, #6413, #575, #9689, #2363, #11468, #11262, #61, #3687, #2063, #6333, #9974, #8429, #6819, #4045, #4521, #5506, #5288, #10288, #63, #52, #1716, #10098, #6457, #8244, #8140, #9876, #5475, #2465, #10042, #2817, #3897, #10570, #7705, #918, #8324, #11211, #1242, #5707, #1530, #10226, #4235, #10711, #6474, #477, #846, #1404, #282, #5416, #9251, #1483, #700, #8060, #11412, #8390, #4323, #11892, #5567, #10892, #6354, #3588, #1061, #5643, #6129, #863, #4714, #6408, #1151, #141, #8440, #1302, #1515, #6604, #2306, #3343 ) ) ;
#4501=ORIENTED_EDGE ( 'NONE', *, *, #1892, .T. ) ;
#4510=DIRECTION ( 'NONE',  ( 0.7071067811865495711, 0.7071067811865455743, 0.000000000000000000 ) ) ;
#4513=CARTESIAN_POINT ( 'NONE',  ( 150.0000000000010800, 15.00000000000008882, -19.99999999999999645 ) ) ;
#4517=CIRCLE ( 'NONE', #740, 75.00000000000001421 ) ;
#4518=EDGE_LOOP ( 'NONE', ( #3054, #11569, #2613, #5394 ) ) ;
#4521=ADVANCED_FACE ( 'NONE', ( #11336 ), #4916, .F. ) ;
#4524=FACE_OUTER_BOUND ( 'NONE', #11676, .T. ) ;
#4529=CARTESIAN_POINT ( 'NONE',  ( 0.000000000000000000, 50.00000000000000000, 0.000000000000000000 ) ) ;
#4530=DIRECTION ( 'NONE',  ( 0.000000000000000000, 1.000000000000000000, -0.000000000000000000 ) ) ;
#4540=ORIENTED_EDGE ( 'NONE', *, *, #8707, .T. ) ;
#4542=VECTOR ( 'NONE', #7423, 1000.000000000000000 ) ;
#4544=EDGE_CURVE ( 'NONE', #3229, #6205, #5728, .T. ) ;
#4555=DIRECTION ( 'NONE',  ( -0.2500000000000003886, 6.938893903907242183E-16, 0.9682458365518542553 ) ) ;
#4559=LINE ( 'NONE', #2749, #8372 ) ;
#4565=CARTESIAN_POINT ( 'NONE',  ( 72.02249449389091751, 49.73282098440206767, 20.92514131019473567 ) ) ;
#4571=CIRCLE ( 'NONE', #10333, 80.00000000000001421 ) ;
#4579=VECTOR ( 'NONE', #11856, 1000.000000000000000 ) ;
#4582=CARTESIAN_POINT ( 'NONE',  ( 142.0710678118665555, 59.99999999999997868, 20.00000000000000000 ) ) ;
#4585=DIRECTION ( 'NONE',  ( 0.000000000000000000, 0.000000000000000000, 1.000000000000000000 ) ) ;
#4591=CIRCLE ( 'NONE', #404, 70.00000000000001421 ) ;
#4592=CARTESIAN_POINT ( 'NONE',  ( 0.9400506840132951680, 15.12220259995254779, 75.00000000000001421 ) ) ;
#4593=ORIENTED_EDGE ( 'NONE', *, *, #5030, .F. ) ;
#4598=CARTESIAN_POINT ( 'NONE',  ( 69.52686081700198883, 19.32205100516523899, -28.12499999881303836 ) ) ;
#4603=CIRCLE ( 'NONE', #2413, 14.99999999999999822 ) ;
#4607=ORIENTED_EDGE ( 'NONE', *, *, #7404, .F. ) ;
#4611=ORIENTED_EDGE ( 'NONE', *, *, #6267, .F. ) ;
#4612=ORIENTED_EDGE ( 'NONE', *, *, #597, .F. ) ;
#4614=ORIENTED_EDGE ( 'NONE', *, *, #8890, .T. ) ;
#4618=DIRECTION ( 'NONE',  ( 0.000000000000000000, 1.000000000000000000, -0.000000000000000000 ) ) ;
#4619=ORIENTED_EDGE ( 'NONE', *, *, #7342, .T. ) ;
#4627=CARTESIAN_POINT ( 'NONE',  ( -15.97595206614365182, 27.41870735413941773, 73.27878722613796469 ) ) ;
#4628=ORIENTED_EDGE ( 'NONE', *, *, #597, .T. ) ;
#4630=DIRECTION ( 'NONE',  ( 0.000000000000000000, 0.000000000000000000, 1.000000000000000000 ) ) ;
#4633=CARTESIAN_POINT ( 'NONE',  ( 0.000000000000000000, 5.000000000000129674, 0.000000000000000000 ) ) ;
#4636=EDGE_CURVE ( 'NONE', #6043, #5183, #3849, .T. ) ;
#4638=DIRECTION ( 'NONE',  ( -0.000000000000000000, -1.000000000000000000, -0.000000000000000000 ) ) ;
#4639=VERTEX_POINT ( 'NONE', #7587 ) ;
#4641=VECTOR ( 'NONE', #6792, 1000.000000000000000 ) ;
#4642=DIRECTION ( 'NONE',  ( 0.000000000000000000, 0.000000000000000000, 1.000000000000000000 ) ) ;
#4645=DIRECTION ( 'NONE',  ( -0.000000000000000000, -1.000000000000000000, -0.000000000000000000 ) ) ;
#4651=VECTOR ( 'NONE', #2400, 1000.000000000000000 ) ;
#4661=CARTESIAN_POINT ( 'NONE',  ( 145.0000000000011369, 225.0000000000000853, 25.00000000000000000 ) ) ;
#4662=DIRECTION ( 'NONE',  ( 0.000000000000000000, 1.000000000000000000, 0.000000000000000000 ) ) ;
#4664=CYLINDRICAL_SURFACE ( 'NONE', #1400, 5.000000000000000888 ) ;
#4667=ORIENTED_EDGE ( 'NONE', *, *, #7495, .T. ) ;
#4668=EDGE_CURVE ( 'NONE', #5411, #2246, #7076, .T. ) ;
#4675=CIRCLE ( 'NONE', #11050, 25.00000000000000000 ) ;
#4680=ORIENTED_EDGE ( 'NONE', *, *, #5783, .T. ) ;
#4685=LINE ( 'NONE', #11306, #206 ) ;
#4690=DIRECTION ( 'NONE',  ( 0.000000000000000000, 1.000000000000000000, 0.000000000000000000 ) ) ;
#4694=PLANE ( 'NONE',  #8860 ) ;
#4706=CIRCLE ( 'NONE', #5309, 75.00000000000001421 ) ;
#4713=EDGE_CURVE ( 'NONE', #4212, #10899, #4973, .T. ) ;
#4714=ADVANCED_FACE ( 'NONE', ( #6094 ), #286, .T. ) ;
#4715=CARTESIAN_POINT ( 'NONE',  ( 74.52821641976538558, 42.10288043194585583, -24.53929266990226665 ) ) ;
#4719=DIRECTION ( 'NONE',  ( 1.000000000000000000, 0.000000000000000000, 0.000000000000000000 ) ) ;
#4720=CARTESIAN_POINT ( 'NONE',  ( 69.91894869711104832, 15.48235109822951472, -27.13685080543958250 ) ) ;
#4738=CIRCLE ( 'NONE', #5747, 3.399999999999999911 ) ;
#4740=ORIENTED_EDGE ( 'NONE', *, *, #10703, .F. ) ;
#4742=EDGE_CURVE ( 'NONE', #1244, #6757, #11267, .T. ) ;
#4746=ORIENTED_EDGE ( 'NONE', *, *, #8736, .F. ) ;
#4750=CARTESIAN_POINT ( 'NONE',  ( 69.72092797052471269, 43.18961593336220517, 27.64057077031492327 ) ) ;
#4751=ORIENTED_EDGE ( 'NONE', *, *, #2050, .T. ) ;
#4754=ORIENTED_EDGE ( 'NONE', *, *, #6785, .T. ) ;
#4757=DIRECTION ( 'NONE',  ( 0.000000000000000000, 0.000000000000000000, -1.000000000000000000 ) ) ;
#4764=EDGE_LOOP ( 'NONE', ( #4667, #10401, #3145, #375 ) ) ;
#4770=DIRECTION ( 'NONE',  ( 0.000000000000000000, 1.000000000000000000, 0.000000000000000000 ) ) ;
#4776=CARTESIAN_POINT ( 'NONE',  ( 70.93011667421792765, 42.07610065776023589, -24.58871393576316677 ) ) ;
#4782=CARTESIAN_POINT ( 'NONE',  ( 71.78382695943247427, 10.51293989489658642, -21.72958296927679456 ) ) ;
#4791=VECTOR ( 'NONE', #11391, 1000.000000000000000 ) ;
#4797=ORIENTED_EDGE ( 'NONE', *, *, #4953, .T. ) ;
#4799=CARTESIAN_POINT ( 'NONE',  ( -20.00000000000000000, 7.965803112215716020, -67.08203932499371547 ) ) ;
#4800=ORIENTED_EDGE ( 'NONE', *, *, #12134, .T. ) ;
#4802=FACE_BOUND ( 'NONE', #6451, .T. ) ;
#4803=AXIS2_PLACEMENT_3D ( 'NONE', #827, #4618, #1698 ) ;
#4814=DIRECTION ( 'NONE',  ( 0.000000000000000000, 0.000000000000000000, -1.000000000000000000 ) ) ;
#4815=CARTESIAN_POINT ( 'NONE',  ( -9.797345851249669835, 17.67135281155243476, 74.36268359007875972 ) ) ;
#4816=ORIENTED_EDGE ( 'NONE', *, *, #1063, .F. ) ;
#4818=CARTESIAN_POINT ( 'NONE',  ( 70.26526821373037990, 13.93439898317257430, 26.22825182065056637 ) ) ;
#4821=CARTESIAN_POINT ( 'NONE',  ( -20.00000000000000355, 50.00000000000000000, -57.08203932499370836 ) ) ;
#4829=DIRECTION ( 'NONE',  ( 0.000000000000000000, -1.000000000000000000, 0.000000000000000000 ) ) ;
#4836=LINE ( 'NONE', #1967, #10072 ) ;
#4837=PLANE ( 'NONE',  #1018 ) ;
#4843=CARTESIAN_POINT ( 'NONE',  ( 71.40110041869772317, 44.02658904323298117, -23.12535642331799579 ) ) ;
#4844=( NAMED_UNIT ( * ) SI_UNIT ( $, .STERADIAN. ) SOLID_ANGLE_UNIT ( ) );
#4849=CARTESIAN_POINT ( 'NONE',  ( 71.89872685388522200, 15.05565339638229716, -21.44363277848739457 ) ) ;
#4856=AXIS2_PLACEMENT_3D ( 'NONE', #10498, #4829, #4642 ) ;
#4857=VECTOR ( 'NONE', #7368, 1000.000000000000000 ) ;
#4860=CARTESIAN_POINT ( 'NONE',  ( 20.00000000000000355, 7.965803112215716020, 57.08203932499370836 ) ) ;
#4871=TOROIDAL_SURFACE ( 'NONE', #1682, 80.00000000000001421, 5.000000000000000000 ) ;
#4880=CARTESIAN_POINT ( 'NONE',  ( -8.467961960366615415, 16.87331863704340762, 74.52176054247227910 ) ) ;
#4882=EDGE_LOOP ( 'NONE', ( #6264, #10031, #6481, #5008 ) ) ;
#4889=FACE_OUTER_BOUND ( 'NONE', #8531, .T. ) ;
#4890=CARTESIAN_POINT ( 'NONE',  ( 72.04250006633355952, 10.25027406420806031, 20.85600298363943494 ) ) ;
#4894=VECTOR ( 'NONE', #1447, 1000.000000000000000 ) ;
#4896=FACE_OUTER_BOUND ( 'NONE', #1156, .T. ) ;
#4897=CARTESIAN_POINT ( 'NONE',  ( 13.80921887069452758, 30.00000000000009237, 73.71774192269630532 ) ) ;
#4899=DIRECTION ( 'NONE',  ( 0.000000000000000000, 1.000000000000000000, 0.000000000000000000 ) ) ;
#4900=AXIS2_PLACEMENT_3D ( 'NONE', #838, #11183, #4630 ) ;
#4901=CARTESIAN_POINT ( 'NONE',  ( 0.000000000000000000, 63.00000000000000000, -57.08203932499371547 ) ) ;
#4911=CARTESIAN_POINT ( 'NONE',  ( 71.54629459846562156, 44.36298584812474388, -22.64784456521648437 ) ) ;
#4915=DIRECTION ( 'NONE',  ( 0.000000000000000000, 0.000000000000000000, 1.000000000000000000 ) ) ;
#4916=PLANE ( 'NONE',  #5476 ) ;
#4917=CARTESIAN_POINT ( 'NONE',  ( 71.40290628601607636, 15.98094810295091861, -23.11746242201430945 ) ) ;
#4926=CARTESIAN_POINT ( 'NONE',  ( 76.77294714683046095, 44.85115178501149558, 21.25082451143517304 ) ) ;
#4932=CARTESIAN_POINT ( 'NONE',  ( 150.0000000000011084, 15.00000000000011724, 20.00000000000000000 ) ) ;
#4941=DIRECTION ( 'NONE',  ( 0.000000000000000000, 1.000000000000000000, 0.000000000000000000 ) ) ;
#4945=AXIS2_PLACEMENT_3D ( 'NONE', #8337, #560, #7300 ) ;
#4953=EDGE_CURVE ( 'NONE', #7931, #9228, #6683, .T. ) ;
#4957=DIRECTION ( 'NONE',  ( 0.000000000000000000, 1.000000000000000000, 0.000000000000000000 ) ) ;
#4958=CARTESIAN_POINT ( 'NONE',  ( 11.76642283301164937, 37.57159100124651729, 74.07168364809568573 ) ) ;
#4960=FACE_OUTER_BOUND ( 'NONE', #4991, .T. ) ;
#4973=LINE ( 'NONE', #7146, #9856 ) ;
#4974=CARTESIAN_POINT ( 'NONE',  ( 76.47662455941971871, 15.31021820271415024, -21.74119912862034454 ) ) ;
#4975=EDGE_LOOP ( 'NONE', ( #1950, #1002, #3909, #9130 ) ) ;
#4980=AXIS2_PLACEMENT_3D ( 'NONE', #4478, #11153, #11651 ) ;
#4982=DIRECTION ( 'NONE',  ( -0.000000000000000000, 1.000000000000000000, -0.000000000000000000 ) ) ;
#4986=CARTESIAN_POINT ( 'NONE',  ( 74.62285592809365653, 42.36573936498655257, 24.41804092124679215 ) ) ;
#4990=DIRECTION ( 'NONE',  ( -1.000000000000000000, -0.000000000000000000, -0.000000000000000000 ) ) ;
#4991=EDGE_LOOP ( 'NONE', ( #11788, #11618, #11193, #2044 ) ) ;
#4992=DIRECTION ( 'NONE',  ( 0.000000000000000000, 0.000000000000000000, -1.000000000000000000 ) ) ;
#5001=CARTESIAN_POINT ( 'NONE',  ( -1.040515751868670957, 14.96447674105763070, 75.00000000000001421 ) ) ;
#5004=DIRECTION ( 'NONE',  ( 0.2499999999999996669, 0.000000000000000000, -0.9682458365518542553 ) ) ;
#5005=CIRCLE ( 'NONE', #3411, 5.000000000000000888 ) ;
#5007=EDGE_CURVE ( 'NONE', #9831, #9708, #6527, .T. ) ;
#5008=ORIENTED_EDGE ( 'NONE', *, *, #3560, .T. ) ;
#5014=EDGE_CURVE ( 'NONE', #10740, #51, #9541, .T. ) ;
#5019=ORIENTED_EDGE ( 'NONE', *, *, #6573, .T. ) ;
#5021=CARTESIAN_POINT ( 'NONE',  ( 3.641433828188992639, 44.20809573012787297, 74.91284009398577837 ) ) ;
#5028=LINE ( 'NONE', #2212, #6787 ) ;
#5030=EDGE_CURVE ( 'NONE', #51, #9490, #2373, .T. ) ;
#5032=DIRECTION ( 'NONE',  ( 1.000000000000000000, 0.000000000000000000, 0.000000000000000000 ) ) ;
#5040=CARTESIAN_POINT ( 'NONE',  ( 74.70253266892970601, 17.45276100714020728, -24.31510929947467048 ) ) ;
#5041=CARTESIAN_POINT ( 'NONE',  ( 70.88057259133860555, 12.10784404089235800, -24.51542725512078391 ) ) ;
#5052=VERTEX_POINT ( 'NONE', #6246 ) ;
#5060=AXIS2_PLACEMENT_3D ( 'NONE', #11769, #1289, #8938 ) ;
#5066=CARTESIAN_POINT ( 'NONE',  ( 0.000000000000000000, 10.00000000000017586, -75.00000000000001421 ) ) ;
#5068=CARTESIAN_POINT ( 'NONE',  ( 145.0000000000011369, 230.0000000000000853, 25.00000000000000000 ) ) ;
#5072=ORIENTED_EDGE ( 'NONE', *, *, #9997, .F. ) ;
#5076=CARTESIAN_POINT ( 'NONE',  ( 75.70742691175847483, 44.06379843619267689, -22.92955197636053555 ) ) ;
#5080=CARTESIAN_POINT ( 'NONE',  ( 71.95699135611712904, 10.32756980217126674, 21.14906888506658333 ) ) ;
#5081=VECTOR ( 'NONE', #6929, 1000.000000000000000 ) ;
#5086=CARTESIAN_POINT ( 'NONE',  ( 7.002289440008276244, 42.59914708353472435, 74.67617861058462836 ) ) ;
#5087=VERTEX_POINT ( 'NONE', #9976 ) ;
#5090=DIRECTION ( 'NONE',  ( 0.000000000000000000, 0.000000000000000000, 1.000000000000000000 ) ) ;
#5099=DIRECTION ( 'NONE',  ( -0.000000000000000000, -1.000000000000000000, -0.000000000000000000 ) ) ;
#5100=LINE ( 'NONE', #8882, #7798 ) ;
#5102=AXIS2_PLACEMENT_3D ( 'NONE', #866, #6536, #8452 ) ;
#5105=FACE_OUTER_BOUND ( 'NONE', #7530, .T. ) ;
#5107=CIRCLE ( 'NONE', #3299, 5.000000000000004441 ) ;
#5108=ORIENTED_EDGE ( 'NONE', *, *, #1673, .T. ) ;
#5111=EDGE_CURVE ( 'NONE', #10790, #9228, #2505, .T. ) ;
#5113=VERTEX_POINT ( 'NONE', #3248 ) ;
#5120=AXIS2_PLACEMENT_3D ( 'NONE', #10299, #8425, #1712 ) ;
#5125=EDGE_CURVE ( 'NONE', #8789, #9381, #9819, .T. ) ;
#5128=CARTESIAN_POINT ( 'NONE',  ( 135.0000000000011084, 67.07106781186550393, 25.00000000000000000 ) ) ;
#5132=CARTESIAN_POINT ( 'NONE',  ( 70.71510656582536569, 12.51027914909978733, 24.99160257227417148 ) ) ;
#5136=CARTESIAN_POINT ( 'NONE',  ( 41.03553390593253170, -41.03553390593296513, -20.00000000000000000 ) ) ;
#5139=ORIENTED_EDGE ( 'NONE', *, *, #9128, .T. ) ;
#5140=CARTESIAN_POINT ( 'NONE',  ( 142.0710678118665555, 59.99999999999998579, -25.00000000000000000 ) ) ;
#5141=CARTESIAN_POINT ( 'NONE',  ( 69.92278643102456215, 15.49627177145660362, 27.12617897809031930 ) ) ;
#5143=CARTESIAN_POINT ( 'NONE',  ( 77.45966692414835109, 15.00000000000008882, 20.00000000000000000 ) ) ;
#5144=CARTESIAN_POINT ( 'NONE',  ( 70.75630133281138967, 47.58060937264504986, -24.87185742758410001 ) ) ;
#5146=CARTESIAN_POINT ( 'NONE',  ( 0.000000000000000000, 110.0000000000000000, 0.000000000000000000 ) ) ;
#5147=CARTESIAN_POINT ( 'NONE',  ( 72.18749001407745425, 45.14382420902206405, 20.39424303846705655 ) ) ;
#5151=EDGE_CURVE ( 'NONE', #8585, #3728, #9339, .T. ) ;
#5153=DIRECTION ( 'NONE',  ( -0.7071067811865486830, -0.7071067811865464625, 0.000000000000000000 ) ) ;
#5160=CARTESIAN_POINT ( 'NONE',  ( 0.000000000000000000, 115.0000000000000000, 0.000000000000000000 ) ) ;
#5162=CARTESIAN_POINT ( 'NONE',  ( -1.041723228171368199, 45.00818216738166910, 74.99454991703274231 ) ) ;
#5166=ORIENTED_EDGE ( 'NONE', *, *, #3603, .F. ) ;
#5176=PLANE ( 'NONE',  #8433 ) ;
#5177=CYLINDRICAL_SURFACE ( 'NONE', #10573, 5.000000000000000888 ) ;
#5183=VERTEX_POINT ( 'NONE', #9400 ) ;
#5185=FACE_OUTER_BOUND ( 'NONE', #9933, .T. ) ;
#5186=ORIENTED_EDGE ( 'NONE', *, *, #10991, .F. ) ;
#5187=CARTESIAN_POINT ( 'NONE',  ( 145.0000000000011369, 0.000000000000000000, -20.00000000000000000 ) ) ;
#5188=DIRECTION ( 'NONE',  ( 0.000000000000000000, 0.000000000000000000, 1.000000000000000000 ) ) ;
#5190=EDGE_CURVE ( 'NONE', #8715, #3552, #823, .T. ) ;
#5192=CARTESIAN_POINT ( 'NONE',  ( 74.16198487095665826, 40.36277934585979210, -25.00000000000000355 ) ) ;
#5194=VECTOR ( 'NONE', #12088, 1000.000000000000000 ) ;
#5197=AXIS2_PLACEMENT_3D ( 'NONE', #3147, #6951, #6019 ) ;
#5198=CARTESIAN_POINT ( 'NONE',  ( 75.47338808840345337, 16.20969531357235027, 23.26499062814251317 ) ) ;
#5200=ORIENTED_EDGE ( 'NONE', *, *, #2952, .T. ) ;
#5206=CARTESIAN_POINT ( 'NONE',  ( 75.38891993288051196, 43.68400779952311552, 23.38442328187086616 ) ) ;
#5212=AXIS2_PLACEMENT_3D ( 'NONE', #5187, #8967, #4362 ) ;
#5216=EDGE_CURVE ( 'NONE', #10965, #4428, #1753, .T. ) ;
#5218=VECTOR ( 'NONE', #7523, 1000.000000000000000 ) ;
#5219=CARTESIAN_POINT ( 'NONE',  ( 0.000000000000000000, 65.00000000000000000, -57.08203932499371547 ) ) ;
#5220=LINE ( 'NONE', #7206, #4443 ) ;
#5225=DIRECTION ( 'NONE',  ( 0.000000000000000000, 0.000000000000000000, 1.000000000000000000 ) ) ;
#5228=ORIENTED_EDGE ( 'NONE', *, *, #3630, .F. ) ;
#5232=ORIENTED_EDGE ( 'NONE', *, *, #1021, .F. ) ;
#5234=CARTESIAN_POINT ( 'NONE',  ( 77.12313347048124967, 15.03062108036313482, -20.63522338802521006 ) ) ;
#5238=CARTESIAN_POINT ( 'NONE',  ( 117.9289321881355193, 45.00000000000008527, 20.00000000000000000 ) ) ;
#5241=CARTESIAN_POINT ( 'NONE',  ( 70.88282142915603856, 47.91395231425131129, -24.51348554696366122 ) ) ;
#5243=ORIENTED_EDGE ( 'NONE', *, *, #10455, .T. ) ;
#5245=CYLINDRICAL_SURFACE ( 'NONE', #6533, 70.00000000000001421 ) ;
#5247=ORIENTED_EDGE ( 'NONE', *, *, #5007, .F. ) ;
#5248=DIRECTION ( 'NONE',  ( -1.000000000000000000, 0.000000000000000000, 0.000000000000000000 ) ) ;
#5252=CARTESIAN_POINT ( 'NONE',  ( 77.45966692414835109, 45.00000000000008527, -20.00000000000000000 ) ) ;
#5257=CARTESIAN_POINT ( 'NONE',  ( 71.02603146012793900, 17.37440083699122795, 24.29862599233017662 ) ) ;
#5266=DIRECTION ( 'NONE',  ( -0.000000000000000000, -1.000000000000000000, -0.000000000000000000 ) ) ;
#5267=CARTESIAN_POINT ( 'NONE',  ( 74.98782882127352423, 43.08750719129150752, 23.93624459205355137 ) ) ;
#5274=EDGE_LOOP ( 'NONE', ( #6173, #9693, #8406, #7181 ) ) ;
#5279=CARTESIAN_POINT ( 'NONE',  ( 72.61843774138908714, 10.00000000000017586, -18.75000000000000000 ) ) ;
#5288=ADVANCED_FACE ( 'NONE', ( #11233 ), #2562, .F. ) ;
#5292=AXIS2_PLACEMENT_3D ( 'NONE', #346, #11831, #4153 ) ;
#5309=AXIS2_PLACEMENT_3D ( 'NONE', #212, #6644, #1905 ) ;
#5310=FACE_OUTER_BOUND ( 'NONE', #3894, .T. ) ;
#5311=DIRECTION ( 'NONE',  ( 1.049727191138621654E-16, 0.5150380749100502698, -0.8571673007021147761 ) ) ;
#5316=ORIENTED_EDGE ( 'NONE', *, *, #2721, .T. ) ;
#5319=CARTESIAN_POINT ( 'NONE',  ( 70.87894850892850229, 18.31681633891911787, 24.74065748999029779 ) ) ;
#5325=ORIENTED_EDGE ( 'NONE', *, *, #6897, .F. ) ;
#5326=CARTESIAN_POINT ( 'NONE',  ( 63.96446609406733330, -63.96446609406769568, 20.00000000000000000 ) ) ;
#5327=FACE_OUTER_BOUND ( 'NONE', #7005, .T. ) ;
#5333=ORIENTED_EDGE ( 'NONE', *, *, #582, .F. ) ;
#5336=FACE_OUTER_BOUND ( 'NONE', #8461, .T. ) ;
#5341=CARTESIAN_POINT ( 'NONE',  ( 1.734723475976807094E-14, 63.00000000000000000, 57.08203932499370836 ) ) ;
#5346=CARTESIAN_POINT ( 'NONE',  ( 69.52686081652184669, 20.00000000000009237, -28.12499999999999645 ) ) ;
#5348=VERTEX_POINT ( 'NONE', #7607 ) ;
#5351=PRODUCT_DEFINITION_FORMATION_WITH_SPECIFIED_SOURCE ( 'ANY', '', #9761, .NOT_KNOWN. ) ;
#5353=ORIENTED_EDGE ( 'NONE', *, *, #2087, .F. ) ;
#5355=ORIENTED_EDGE ( 'NONE', *, *, #6897, .T. ) ;
#5359=DIRECTION ( 'NONE',  ( -0.7071067811865454633, 0.7071067811865495711, 0.000000000000000000 ) ) ;
#5362=CARTESIAN_POINT ( 'NONE',  ( 69.90350624952219505, 44.39669317652923297, -27.17578603812305360 ) ) ;
#5372=VERTEX_POINT ( 'NONE', #1191 ) ;
#5373=DIRECTION ( 'NONE',  ( 0.000000000000000000, 0.000000000000000000, 1.000000000000000000 ) ) ;
#5376=VERTEX_POINT ( 'NONE', #3993 ) ;
#5380=AXIS2_PLACEMENT_3D ( 'NONE', #4010, #2886, #6695 ) ;
#5383=DIRECTION ( 'NONE',  ( 0.000000000000000000, -1.000000000000000000, -0.000000000000000000 ) ) ;
#5384=DIRECTION ( 'NONE',  ( 0.000000000000000000, 1.000000000000000000, 0.000000000000000000 ) ) ;
#5386=CYLINDRICAL_SURFACE ( 'NONE', #6652, 4.999999999999997335 ) ;
#5387=CARTESIAN_POINT ( 'NONE',  ( 70.67711243716091474, 47.36801559909221737, 25.09579365358156622 ) ) ;
#5388=VERTEX_POINT ( 'NONE', #2936 ) ;
#5394=ORIENTED_EDGE ( 'NONE', *, *, #9547, .F. ) ;
#5399=STYLED_ITEM ( 'NONE', ( #11456 ), #10022 ) ;
#5403=EDGE_CURVE ( 'NONE', #6450, #9081, #8655, .T. ) ;
#5409=LINE ( 'NONE', #2594, #4404 ) ;
#5411=VERTEX_POINT ( 'NONE', #11665 ) ;
#5416=ADVANCED_FACE ( 'NONE', ( #1006 ), #11483, .T. ) ;
#5420=DIRECTION ( 'NONE',  ( 0.000000000000000000, 0.000000000000000000, -1.000000000000000000 ) ) ;
#5421=CARTESIAN_POINT ( 'NONE',  ( 117.9289321881355193, 50.00000000000008527, -19.99999999999999645 ) ) ;
#5424=DIRECTION ( 'NONE',  ( 0.000000000000000000, 1.000000000000000000, 0.000000000000000000 ) ) ;
#5429=AXIS2_PLACEMENT_3D ( 'NONE', #3587, #6396, #1596 ) ;
#5432=ORIENTED_EDGE ( 'NONE', *, *, #3831, .F. ) ;
#5434=DIRECTION ( 'NONE',  ( -1.000000000000000000, 0.000000000000000000, 3.469446951953613203E-16 ) ) ;
#5454=ORIENTED_EDGE ( 'NONE', *, *, #6310, .F. ) ;
#5459=EDGE_LOOP ( 'NONE', ( #847, #4501, #2660, #9047, #4797, #7533, #3721 ) ) ;
#5468=CARTESIAN_POINT ( 'NONE',  ( 12.60805306350328969, 24.10018532896172516, 73.93285131058543413 ) ) ;
#5471=B_SPLINE_CURVE_WITH_KNOTS ( 'NONE', 3,
 ( #7409, #4592, #11086, #10317, #2722, #2542, #1608, #7468, #6531, #1787, #5600, #3472, #472, #4399, #4281, #10008, #736, #7338, #5468, #8194, #1602, #9252, #8073, #12084, #10066, #9123 ),
 .UNSPECIFIED., .F., .F.,
 ( 4, 2, 2, 2, 2, 2, 2, 2, 2, 2, 2, 2, 4 ),
 ( 1.022432916270031883E-18, 0.002788363146399075020, 0.004182544719598612314, 0.005576726292798150041, 0.008365089439197226362, 0.009759271012396762354, 0.01115345258559629835, 0.01394181573199535992, 0.01533599730519489591, 0.01673017887839442844, 0.01951854202479350042, 0.02091272359799303121, 0.02230690517119256200 ),
 .UNSPECIFIED. ) ;
#5475=ADVANCED_FACE ( 'NONE', ( #4802, #8592 ), #53, .T. ) ;
#5476=AXIS2_PLACEMENT_3D ( 'NONE', #7712, #98, #10389 ) ;
#5478=CIRCLE ( 'NONE', #8047, 5.000000000000000888 ) ;
#5481=PLANE ( 'NONE',  #5102 ) ;
#5485=EDGE_CURVE ( 'NONE', #298, #5411, #6851, .T. ) ;
#5487=VERTEX_POINT ( 'NONE', #1249 ) ;
#5492=CARTESIAN_POINT ( 'NONE',  ( 0.000000000000000000, 115.0000000000000000, -15.00000000000000000 ) ) ;
#5493=DIRECTION ( 'NONE',  ( 0.000000000000000000, 0.000000000000000000, -1.000000000000000000 ) ) ;
#5502=AXIS2_PLACEMENT_3D ( 'NONE', #11414, #6323, #12063 ) ;
#5506=ADVANCED_FACE ( 'NONE', ( #11790 ), #5176, .F. ) ;
#5510=APPLICATION_CONTEXT ( 'automotive_design' ) ;
#5512=VECTOR ( 'NONE', #149, 1000.000000000000000 ) ;
#5515=CARTESIAN_POINT ( 'NONE',  ( 145.0000000000011369, 67.07106781186550393, -25.00000000000000000 ) ) ;
#5518=CARTESIAN_POINT ( 'NONE',  ( 72.45821416003295212, 45.13374170404204477, 19.37058730516574556 ) ) ;
#5526=ORIENTED_EDGE ( 'NONE', *, *, #2952, .F. ) ;
#5527=CARTESIAN_POINT ( 'NONE',  ( 13.80921887069452758, 30.00000000000009237, 75.00000000000001421 ) ) ;
#5533=CARTESIAN_POINT ( 'NONE',  ( -15.63374382699839948, 34.08284429348438493, 73.35265631139654374 ) ) ;
#5540=EDGE_CURVE ( 'NONE', #298, #5087, #10961, .T. ) ;
#5544=CARTESIAN_POINT ( 'NONE',  ( 69.52686081652184669, 20.00000000000008882, -28.12499999999999645 ) ) ;
#5545=ORIENTED_EDGE ( 'NONE', *, *, #10347, .T. ) ;
#5547=FACE_OUTER_BOUND ( 'NONE', #7793, .T. ) ;
#5554=ORIENTED_EDGE ( 'NONE', *, *, #6608, .F. ) ;
#5557=EDGE_LOOP ( 'NONE', ( #1710, #11906, #8241, #11166 ) ) ;
#5567=ADVANCED_FACE ( 'NONE', ( #8836 ), #9958, .T. ) ;
#5575=CARTESIAN_POINT ( 'NONE',  ( 145.0000000000011369, 30.00000000000008882, 20.00000000000000000 ) ) ;
#5582=DIRECTION ( 'NONE',  ( 1.000000000000000000, -0.000000000000000000, 1.564230817409691233E-15 ) ) ;
#5585=AXIS2_PLACEMENT_3D ( 'NONE', #2733, #6421, #752 ) ;
#5595=CARTESIAN_POINT ( 'NONE',  ( 8.572527594031474570E-15, -10.00000000000000000, -70.00000000000001421 ) ) ;
#5600=CARTESIAN_POINT ( 'NONE',  ( 8.486113780751869839, 18.52929026929728451, 74.51918556699330054 ) ) ;
#5604=AXIS2_PLACEMENT_3D ( 'NONE', #10163, #10348, #10097 ) ;
#5607=DIRECTION ( 'NONE',  ( 0.000000000000000000, 1.000000000000000000, 0.000000000000000000 ) ) ;
#5618=DIRECTION ( 'NONE',  ( -1.000000000000000000, 0.000000000000000000, 0.000000000000000000 ) ) ;
#5621=VECTOR ( 'NONE', #1998, 1000.000000000000000 ) ;
#5634=CARTESIAN_POINT ( 'NONE',  ( 0.000000000000000000, -10.00000000000000000, 0.000000000000000000 ) ) ;
#5637=DIRECTION ( 'NONE',  ( 0.000000000000000000, -0.000000000000000000, 1.000000000000000000 ) ) ;
#5643=ADVANCED_FACE ( 'NONE', ( #5547 ), #3547, .T. ) ;
#5652=CARTESIAN_POINT ( 'NONE',  ( 69.52686081652184669, 40.00000000000009237, 28.12499999999999645 ) ) ;
#5653=DIRECTION ( 'NONE',  ( 0.000000000000000000, 0.000000000000000000, 1.000000000000000000 ) ) ;
#5655=CARTESIAN_POINT ( 'NONE',  ( -10.99915987420040864, 41.36037153982223202, 74.19004793912918672 ) ) ;
#5658=DIRECTION ( 'NONE',  ( 0.7071067811865447972, -0.7071067811865503483, 0.000000000000000000 ) ) ;
#5660=CARTESIAN_POINT ( 'NONE',  ( 71.06140945338827919, 42.80295775297188499, -24.19089746873602209 ) ) ;
#5667=CARTESIAN_POINT ( 'NONE',  ( 74.18968745904427919, 19.32840679882189860, -24.96588476870653395 ) ) ;
#5685=CARTESIAN_POINT ( 'NONE',  ( 138.5355339059338462, 63.53553390593273775, 25.00000000000000000 ) ) ;
#5690=MECHANICAL_DESIGN_GEOMETRIC_PRESENTATION_REPRESENTATION('',(#2896),#9448);
#5692=VECTOR ( 'NONE', #4719, 1000.000000000000000 ) ;
#5695=DIRECTION ( 'NONE',  ( 0.000000000000000000, 1.000000000000000000, 0.000000000000000000 ) ) ;
#5702=DIRECTION ( 'NONE',  ( 0.000000000000000000, 0.000000000000000000, 1.000000000000000000 ) ) ;
#5707=ADVANCED_FACE ( 'NONE', ( #2549 ), #4414, .T. ) ;
#5714=DIRECTION ( 'NONE',  ( 0.000000000000000000, 0.000000000000000000, 1.000000000000000000 ) ) ;
#5715=DIRECTION ( 'NONE',  ( 0.000000000000000000, 0.000000000000000000, 1.000000000000000000 ) ) ;
#5718=CARTESIAN_POINT ( 'NONE',  ( 145.0000000000011369, 225.0000000000000853, -20.00000000000000000 ) ) ;
#5722=CARTESIAN_POINT ( 'NONE',  ( 71.99568681135052373, 45.03885011699624386, -21.09760594592234284 ) ) ;
#5728=LINE ( 'NONE', #11398, #5692 ) ;
#5729=CARTESIAN_POINT ( 'NONE',  ( 71.69660397288473064, 15.34952436719795621, -22.14258685050887365 ) ) ;
#5733=ORIENTED_EDGE ( 'NONE', *, *, #2906, .T. ) ;
#5745=DIRECTION ( 'NONE',  ( 0.000000000000000000, -1.000000000000000000, 0.000000000000000000 ) ) ;
#5747=AXIS2_PLACEMENT_3D ( 'NONE', #8843, #1501, #11918 ) ;
#5749=EDGE_LOOP ( 'NONE', ( #2154, #10631, #6381, #11929 ) ) ;
#5757=FACE_OUTER_BOUND ( 'NONE', #3793, .T. ) ;
#5763=LINE ( 'NONE', #9542, #7303 ) ;
#5767=FACE_OUTER_BOUND ( 'NONE', #7957, .T. ) ;
#5768=ORIENTED_EDGE ( 'NONE', *, *, #9964, .F. ) ;
#5771=CARTESIAN_POINT ( 'NONE',  ( -20.00000000000004263, 54.99999999999999289, 67.08203932499370126 ) ) ;
#5772=CARTESIAN_POINT ( 'NONE',  ( 0.000000000000000000, 115.0000000000000000, 3.399999999999999911 ) ) ;
#5774=CARTESIAN_POINT ( 'NONE',  ( 20.00000000000000355, 63.00000000000000000, 57.08203932499370836 ) ) ;
#5775=AXIS2_PLACEMENT_3D ( 'NONE', #4190, #7812, #7922 ) ;
#5776=AXIS2_PLACEMENT_3D ( 'NONE', #1139, #11616, #4000 ) ;
#5777=DIRECTION ( 'NONE',  ( -0.000000000000000000, 1.000000000000000000, -0.000000000000000000 ) ) ;
#5778=( BOUNDED_CURVE ( )  B_SPLINE_CURVE ( 3, ( #2698, #4442, #8303, #10297 ),
 .UNSPECIFIED., .F., .F. ) 
 B_SPLINE_CURVE_WITH_KNOTS ( ( 4, 4 ),
 ( 1.860548028230944562, 2.013707370868536461 ),
 .UNSPECIFIED. ) 
 CURVE ( )  GEOMETRIC_REPRESENTATION_ITEM ( )  RATIONAL_B_SPLINE_CURVE ( ( 1.000000000000000000, 0.9980461397859388128, 0.9980461397859388128, 1.000000000000000000 ) ) 
 REPRESENTATION_ITEM ( '' )  );
#5780=FACE_OUTER_BOUND ( 'NONE', #3979, .T. ) ;
#5781=SHAPE_REPRESENTATION_RELATIONSHIP ( 'NONE' , 'NONE' ,  #9674, #10022 ) ;
#5783=EDGE_CURVE ( 'NONE', #357, #4020, #484, .T. ) ;
#5784=CARTESIAN_POINT ( 'NONE',  ( 71.26020304811987671, 48.71088408138511738, -23.39373652035234841 ) ) ;
#5786=DIRECTION ( 'NONE',  ( 0.000000000000000000, 1.000000000000000000, 0.000000000000000000 ) ) ;
#5788=CARTESIAN_POINT ( 'NONE',  ( 75.74050859682202486, 15.90871218390771347, -22.87883167916282900 ) ) ;
#5797=EDGE_LOOP ( 'NONE', ( #8122, #1171, #2144, #2319 ) ) ;
#5799=CARTESIAN_POINT ( 'NONE',  ( 74.75199569173395275, 42.65375252791112359, 24.25052255086779951 ) ) ;
#5803=ORIENTED_EDGE ( 'NONE', *, *, #11643, .T. ) ;
#5804=DIRECTION ( 'NONE',  ( -0.7071067811865495711, -0.7071067811865455743, -0.000000000000000000 ) ) ;
#5815=DIRECTION ( 'NONE',  ( -0.000000000000000000, -1.000000000000000000, -0.000000000000000000 ) ) ;
#5818=CARTESIAN_POINT ( 'NONE',  ( 69.52686081652183248, 19.67220229193595316, 28.12500000000000355 ) ) ;
#5823=DIRECTION ( 'NONE',  ( -0.000000000000000000, 1.000000000000000000, -0.000000000000000000 ) ) ;
#5832=CARTESIAN_POINT ( 'NONE',  ( 165.0000000000011369, 37.07106781186553945, 25.00000000000000000 ) ) ;
#5836=CARTESIAN_POINT ( 'NONE',  ( 75.00000000000001421, 45.00000000000008527, 25.00000000000000000 ) ) ;
#5840=ORIENTED_EDGE ( 'NONE', *, *, #9998, .T. ) ;
#5842=CARTESIAN_POINT ( 'NONE',  ( 70.10024745330821361, 45.37027644699535500, -26.66438925502398760 ) ) ;
#5850=DIRECTION ( 'NONE',  ( -0.000000000000000000, -0.000000000000000000, 1.000000000000000000 ) ) ;
#5852=EDGE_CURVE ( 'NONE', #4428, #4212, #10433, .T. ) ;
#5856=VECTOR ( 'NONE', #1367, 1000.000000000000000 ) ;
#5859=CARTESIAN_POINT ( 'NONE',  ( 76.23530124607874825, 44.53425327553449620, 22.12995508525856891 ) ) ;
#5862=DIRECTION ( 'NONE',  ( 0.000000000000000000, -1.000000000000000000, 0.000000000000000000 ) ) ;
#5868=VECTOR ( 'NONE', #10170, 1000.000000000000000 ) ;
#5876=CARTESIAN_POINT ( 'NONE',  ( -2.075489372555320955, 14.99018364498190969, 74.97835631650174548 ) ) ;
#5879=AXIS2_PLACEMENT_3D ( 'NONE', #9600, #5935, #3187 ) ;
#5882=VERTEX_POINT ( 'NONE', #2921 ) ;
#5889=CARTESIAN_POINT ( 'NONE',  ( 0.000000000000000000, 0.000000000000000000, -25.00000000000000000 ) ) ;
#5894=CARTESIAN_POINT ( 'NONE',  ( 9.450654096908945471E-15, 44.95265997413478942, 75.00000000000001421 ) ) ;
#5908=DIRECTION ( 'NONE',  ( 0.000000000000000000, -0.000000000000000000, 1.000000000000000000 ) ) ;
#5910=CARTESIAN_POINT ( 'NONE',  ( 71.95778018440435631, 10.32676784893601862, -21.14640536576783347 ) ) ;
#5913=DIRECTION ( 'NONE',  ( -0.000000000000000000, -1.000000000000000000, -0.000000000000000000 ) ) ;
#5924=CARTESIAN_POINT ( 'NONE',  ( 70.71067811865476926, 20.00000000000009237, -25.00000000000000000 ) ) ;
#5928=ORIENTED_EDGE ( 'NONE', *, *, #1622, .T. ) ;
#5932=ADVANCED_FACE ( 'NONE', ( #5105 ), #3100, .T. ) ;
#5933=ADVANCED_FACE ( 'NONE', ( #3160 ), #8634, .T. ) ;
#5935=DIRECTION ( 'NONE',  ( -1.000000000000000000, 0.000000000000000000, 0.000000000000000000 ) ) ;
#5938=CARTESIAN_POINT ( 'NONE',  ( 69.57537924859245493, 18.37100271180785072, 28.00483409347995689 ) ) ;
#5942=CARTESIAN_POINT ( 'NONE',  ( 77.12362621866023460, 44.96938750309810473, -20.63427607811778230 ) ) ;
#5944=DIRECTION ( 'NONE',  ( -0.000000000000000000, -1.000000000000000000, -0.000000000000000000 ) ) ;
#5953=DIRECTION ( 'NONE',  ( 0.000000000000000000, 0.000000000000000000, 1.000000000000000000 ) ) ;
#5954=CARTESIAN_POINT ( 'NONE',  ( 12.60718874148162705, 35.90182366188934537, 73.93299872726009880 ) ) ;
#5956=DIRECTION ( 'NONE',  ( 0.000000000000000000, 0.000000000000000000, 1.000000000000000000 ) ) ;
#5957=CARTESIAN_POINT ( 'NONE',  ( 1.088204915335219061E-15, 15.04734002586538821, 75.00000000000001421 ) ) ;
#5960=LINE ( 'NONE', #1163, #4791 ) ;
#5964=DIRECTION ( 'NONE',  ( -1.000000000000000000, 0.000000000000000000, -0.000000000000000000 ) ) ;
#5968=CARTESIAN_POINT ( 'NONE',  ( 72.61843774138908714, 15.00000000000009237, -18.74999999999999645 ) ) ;
#5973=VECTOR ( 'NONE', #7981, 1000.000000000000000 ) ;
#5978=AXIS2_PLACEMENT_3D ( 'NONE', #964, #5944, #4757 ) ;
#5982=FACE_OUTER_BOUND ( 'NONE', #10395, .T. ) ;
#5994=VERTEX_POINT ( 'NONE', #6096 ) ;
#5996=FACE_OUTER_BOUND ( 'NONE', #5749, .T. ) ;
#5999=CARTESIAN_POINT ( 'NONE',  ( 72.45442684796221045, 10.00000000000009415, 19.38521145883884955 ) ) ;
#6003=CARTESIAN_POINT ( 'NONE',  ( 76.77549258727734127, 44.85216755992210125, -21.24643021050508196 ) ) ;
#6005=VERTEX_POINT ( 'NONE', #11900 ) ;
#6008=EDGE_CURVE ( 'NONE', #5411, #1747, #8942, .T. ) ;
#6011=ORIENTED_EDGE ( 'NONE', *, *, #7796, .T. ) ;
#6012=CARTESIAN_POINT ( 'NONE',  ( 74.16198487095665826, 19.63722065414038553, 25.00000000000000355 ) ) ;
#6019=DIRECTION ( 'NONE',  ( -1.000000000000000000, 0.000000000000000000, -0.000000000000000000 ) ) ;
#6024=EDGE_CURVE ( 'NONE', #9442, #7980, #9759, .T. ) ;
#6026=VERTEX_POINT ( 'NONE', #2407 ) ;
#6032=EDGE_CURVE ( 'NONE', #7410, #9178, #8551, .T. ) ;
#6033=CARTESIAN_POINT ( 'NONE',  ( 71.75476781871512344, 10.54753387286905664, -21.82544253889692953 ) ) ;
#6043=VERTEX_POINT ( 'NONE', #10126 ) ;
#6056=CARTESIAN_POINT ( 'NONE',  ( -12.78987254884215652, 20.47477440642036939, 73.90223226960110026 ) ) ;
#6059=CARTESIAN_POINT ( 'NONE',  ( 72.61843774138907293, 10.00000000000017586, 18.75000000000000000 ) ) ;
#6066=CARTESIAN_POINT ( 'NONE',  ( 70.79540202493410561, 19.57470310065012953, 24.98706380095428159 ) ) ;
#6071=CARTESIAN_POINT ( 'NONE',  ( 74.21645788709501801, 40.83568806828487396, -24.93253696209796644 ) ) ;
#6074=CARTESIAN_POINT ( 'NONE',  ( 71.00672680945956472, 48.18257563199676952, 24.14780939829461204 ) ) ;
#6079=CYLINDRICAL_SURFACE ( 'NONE', #11543, 3.399999999999999911 ) ;
#6081=DIRECTION ( 'NONE',  ( -0.000000000000000000, 1.000000000000000000, -0.000000000000000000 ) ) ;
#6083=AXIS2_PLACEMENT_3D ( 'NONE', #7243, #10091, #5373 ) ;
#6086=ORIENTED_EDGE ( 'NONE', *, *, #7895, .T. ) ;
#6093=VECTOR ( 'NONE', #5607, 1000.000000000000000 ) ;
#6094=FACE_OUTER_BOUND ( 'NONE', #9527, .T. ) ;
#6096=CARTESIAN_POINT ( 'NONE',  ( -16.19078112930547064, 30.00000000000008882, 65.00000000000000000 ) ) ;
#6106=CARTESIAN_POINT ( 'NONE',  ( 77.29386075506076281, 45.00000000000009237, 20.32108226578738197 ) ) ;
#6109=DIRECTION ( 'NONE',  ( -0.7071067811865437980, 0.7071067811865513475, 0.000000000000000000 ) ) ;
#6112=CARTESIAN_POINT ( 'NONE',  ( 77.45966692414835109, 15.00000000000008882, -19.99999999999999645 ) ) ;
#6114=CARTESIAN_POINT ( 'NONE',  ( 70.26526821373037990, 46.06560101682759978, -26.22825182065055927 ) ) ;
#6119=CYLINDRICAL_SURFACE ( 'NONE', #8777, 15.00000000000000000 ) ;
#6127=EDGE_CURVE ( 'NONE', #5052, #9708, #3658, .T. ) ;
#6128=CARTESIAN_POINT ( 'NONE',  ( 74.52821641976770195, 17.89711956805382442, 24.53929266990205704 ) ) ;
#6129=ADVANCED_FACE ( 'NONE', ( #4134 ), #10554, .F. ) ;
#6131=CARTESIAN_POINT ( 'NONE',  ( 71.95699135611761221, 49.67243019782949887, -21.14906888506497751 ) ) ;
#6135=CARTESIAN_POINT ( 'NONE',  ( 70.30108951986187549, 46.17501438243731116, 26.13045860990727931 ) ) ;
#6136=ORIENTED_EDGE ( 'NONE', *, *, #3756, .F. ) ;
#6143=EDGE_LOOP ( 'NONE', ( #3324, #12035, #11210, #2971 ) ) ;
#6146=CARTESIAN_POINT ( 'NONE',  ( 0.000000000000000000, 50.00000000000000000, 0.000000000000000000 ) ) ;
#6150=DIRECTION ( 'NONE',  ( -0.000000000000000000, -0.000000000000000000, 1.000000000000000000 ) ) ;
#6152=CARTESIAN_POINT ( 'NONE',  ( 72.02249449389087488, 10.26717901559811175, -20.92514131019472146 ) ) ;
#6157=CIRCLE ( 'NONE', #4360, 10.00000000000000888 ) ;
#6160=ORIENTED_EDGE ( 'NONE', *, *, #9074, .T. ) ;
#6170=ORIENTED_EDGE ( 'NONE', *, *, #9305, .F. ) ;
#6173=ORIENTED_EDGE ( 'NONE', *, *, #8858, .F. ) ;
#6175=DIRECTION ( 'NONE',  ( -1.000000000000000000, 4.163336342344333082E-15, 0.000000000000000000 ) ) ;
#6183=LINE ( 'NONE', #8163, #2612 ) ;
#6184=CIRCLE ( 'NONE', #9758, 3.399999999999999911 ) ;
#6188=CARTESIAN_POINT ( 'NONE',  ( 70.67517779188629845, 12.63729133232783219, 25.10124566575549565 ) ) ;
#6191=CARTESIAN_POINT ( 'NONE',  ( 74.31677170407374433, 18.58020549109977892, 24.80746953044373626 ) ) ;
#6197=CARTESIAN_POINT ( 'NONE',  ( 70.93313137955965431, 42.06848318385853247, 24.57887570927810472 ) ) ;
#6205=VERTEX_POINT ( 'NONE', #646 ) ;
#6206=ORIENTED_EDGE ( 'NONE', *, *, #9732, .T. ) ;
#6210=CARTESIAN_POINT ( 'NONE',  ( 117.9289321881355193, 40.00000000000009237, 25.00000000000000000 ) ) ;
#6211=CIRCLE ( 'NONE', #234, 65.00000000000001421 ) ;
#6213=CARTESIAN_POINT ( 'NONE',  ( 1.836970198721029589E-15, 115.0000000000000000, 15.00000000000000000 ) ) ;
#6220=CARTESIAN_POINT ( 'NONE',  ( -20.00000000000000355, 54.99999999999999289, 57.08203932499370836 ) ) ;
#6222=VECTOR ( 'NONE', #9991, 1000.000000000000000 ) ;
#6224=CARTESIAN_POINT ( 'NONE',  ( 77.45966692414835109, 45.00000000000008527, 20.00000000000000000 ) ) ;
#6226=CARTESIAN_POINT ( 'NONE',  ( 77.45966692414835109, 45.00000000000008527, 20.00000000000000000 ) ) ;
#6227=CARTESIAN_POINT ( 'NONE',  ( 74.40419232661420779, 18.25469906876584147, -24.69784343973813989 ) ) ;
#6229=AXIS2_PLACEMENT_3D ( 'NONE', #3310, #9148, #7048 ) ;
#6235=CARTESIAN_POINT ( 'NONE',  ( 69.52686081652183248, 40.32779770806423159, -28.12499999999998934 ) ) ;
#6236=VECTOR ( 'NONE', #2367, 1000.000000000000000 ) ;
#6238=DIRECTION ( 'NONE',  ( 0.000000000000000000, 0.000000000000000000, 1.000000000000000000 ) ) ;
#6243=DIRECTION ( 'NONE',  ( 0.000000000000000000, 1.000000000000000000, 0.000000000000000000 ) ) ;
#6246=CARTESIAN_POINT ( 'NONE',  ( 77.45966692414835109, 15.00000000000008882, 20.00000000000000000 ) ) ;
#6252=CARTESIAN_POINT ( 'NONE',  ( 74.37657609242243950, 18.35338373004630341, 24.73263046052399972 ) ) ;
#6255=CARTESIAN_POINT ( 'NONE',  ( 76.59657895567488595, 15.23512201424183843, 21.54700147973310820 ) ) ;
#6261=CARTESIAN_POINT ( 'NONE',  ( 70.03362437693273534, 45.09447798584402989, 26.84082993662288175 ) ) ;
#6264=ORIENTED_EDGE ( 'NONE', *, *, #8272, .T. ) ;
#6267=EDGE_CURVE ( 'NONE', #9708, #6555, #5478, .T. ) ;
#6268=UNCERTAINTY_MEASURE_WITH_UNIT (LENGTH_MEASURE( 1.000000000000000082E-05 ), #10444, 'distance_accuracy_value', 'NONE');
#6285=CARTESIAN_POINT ( 'NONE',  ( 74.16198487095665826, 20.00000000000009237, 25.00000000000000000 ) ) ;
#6286=ORIENTED_EDGE ( 'NONE', *, *, #854, .F. ) ;
#6290=CARTESIAN_POINT ( 'NONE',  ( 76.59271415824169082, 15.23730819188808283, -21.55336028430495787 ) ) ;
#6296=CARTESIAN_POINT ( 'NONE',  ( 69.52686081652184669, 40.00000000000009237, -28.12499999999999645 ) ) ;
#6310=EDGE_CURVE ( 'NONE', #737, #9831, #9226, .T. ) ;
#6321=CARTESIAN_POINT ( 'NONE',  ( 70.88237045016090576, 41.67245225087944505, 24.73035864412370799 ) ) ;
#6323=DIRECTION ( 'NONE',  ( 1.000000000000000000, 0.000000000000000000, 0.000000000000000000 ) ) ;
#6327=EDGE_CURVE ( 'NONE', #10619, #7679, #2908, .T. ) ;
#6333=ADVANCED_FACE ( 'NONE', ( #5757 ), #6686, .T. ) ;
#6339=( BOUNDED_CURVE ( )  B_SPLINE_CURVE ( 3, ( #7794, #11611, #3060, #7165 ),
 .UNSPECIFIED., .F., .F. ) 
 B_SPLINE_CURVE_WITH_KNOTS ( ( 4, 4 ),
 ( 0.000000000000000000, 1.570796326794895448 ),
 .UNSPECIFIED. ) 
 CURVE ( )  GEOMETRIC_REPRESENTATION_ITEM ( )  RATIONAL_B_SPLINE_CURVE ( ( 1.000000000000000000, 0.8047378541243652705, 0.8047378541243652705, 1.000000000000000000 ) ) 
 REPRESENTATION_ITEM ( '' )  );
#6350=CARTESIAN_POINT ( 'NONE',  ( 74.19368986856427739, 19.28333586514525777, -24.96097029013992241 ) ) ;
#6354=ADVANCED_FACE ( 'NONE', ( #3751 ), #10043, .F. ) ;
#6359=CARTESIAN_POINT ( 'NONE',  ( 0.000000000000000000, 109.0000000000000000, 3.399999999999999911 ) ) ;
#6378=VERTEX_POINT ( 'NONE', #5515 ) ;
#6379=DIRECTION ( 'NONE',  ( 0.000000000000000000, 1.000000000000000000, 0.000000000000000000 ) ) ;
#6381=ORIENTED_EDGE ( 'NONE', *, *, #8252, .F. ) ;
#6384=VERTEX_POINT ( 'NONE', #1946 ) ;
#6385=LINE ( 'NONE', #4799, #4422 ) ;
#6387=CARTESIAN_POINT ( 'NONE',  ( 9.184850993605150311E-15, 10.00000000000017586, -75.00000000000001421 ) ) ;
#6395=EDGE_CURVE ( 'NONE', #3340, #2354, #3511, .T. ) ;
#6396=DIRECTION ( 'NONE',  ( -0.000000000000000000, -0.000000000000000000, 1.000000000000000000 ) ) ;
#6400=VECTOR ( 'NONE', #9156, 1000.000000000000000 ) ;
#6401=DIRECTION ( 'NONE',  ( -1.000000000000000000, 0.000000000000000000, 0.000000000000000000 ) ) ;
#6403=CARTESIAN_POINT ( 'NONE',  ( 69.52686081652187511, 19.34506120843814614, -28.12500000000000000 ) ) ;
#6408=ADVANCED_FACE ( 'NONE', ( #5996 ), #254, .T. ) ;
#6412=EDGE_CURVE ( 'NONE', #10667, #298, #11730, .T. ) ;
#6413=ADVANCED_FACE ( 'NONE', ( #11675 ), #8788, .T. ) ;
#6416=CARTESIAN_POINT ( 'NONE',  ( 74.30294665491157957, 18.67686843580081302, -24.82467190422460845 ) ) ;
#6417=VERTEX_POINT ( 'NONE', #2944 ) ;
#6420=ORIENTED_EDGE ( 'NONE', *, *, #7403, .T. ) ;
#6421=DIRECTION ( 'NONE',  ( 1.000000000000000000, -0.000000000000000000, -0.000000000000000000 ) ) ;
#6429=DIRECTION ( 'NONE',  ( 0.2500000000000003886, 6.938893903907242183E-16, 0.9682458365518542553 ) ) ;
#6430=CARTESIAN_POINT ( 'NONE',  ( -20.00000000000000355, 7.965803112215716020, 57.08203932499370836 ) ) ;
#6432=DIRECTION ( 'NONE',  ( 0.7071067811865513475, 0.7071067811865437980, -0.000000000000000000 ) ) ;
#6434=CARTESIAN_POINT ( 'NONE',  ( 72.61843774138907293, 50.00000000000000000, 18.75000000000000000 ) ) ;
#6439=EDGE_CURVE ( 'NONE', #9777, #5376, #6987, .T. ) ;
#6445=CARTESIAN_POINT ( 'NONE',  ( -20.00000000000000355, 7.965803112215716020, 57.08203932499370836 ) ) ;
#6450=VERTEX_POINT ( 'NONE', #4064 ) ;
#6451=EDGE_LOOP ( 'NONE', ( #11605, #2728 ) ) ;
#6453=VECTOR ( 'NONE', #2026, 1000.000000000000000 ) ;
#6457=ADVANCED_FACE ( 'NONE', ( #1074 ), #128, .F. ) ;
#6462=CARTESIAN_POINT ( 'NONE',  ( -2.076303083421399354, 44.98277681526300853, 74.97303962124122734 ) ) ;
#6463=CARTESIAN_POINT ( 'NONE',  ( 0.000000000000000000, 65.00000000000000000, 0.000000000000000000 ) ) ;
#6467=DIRECTION ( 'NONE',  ( -0.000000000000000000, -1.000000000000000000, -0.000000000000000000 ) ) ;
#6468=EDGE_CURVE ( 'NONE', #8398, #8933, #2284, .T. ) ;
#6470=LINE ( 'NONE', #12090, #5218 ) ;
#6474=ADVANCED_FACE ( 'NONE', ( #10666 ), #2069, .T. ) ;
#6481=ORIENTED_EDGE ( 'NONE', *, *, #8736, .T. ) ;
#6486=EDGE_LOOP ( 'NONE', ( #6206, #4628, #8800, #8607, #2421 ) ) ;
#6497=AXIS2_PLACEMENT_3D ( 'NONE', #4291, #6109, #12094 ) ;
#6499=LINE ( 'NONE', #11359, #4208 ) ;
#6506=CARTESIAN_POINT ( 'NONE',  ( -20.00000000000000000, 54.99999999999999289, 67.08203932499370126 ) ) ;
#6507=CARTESIAN_POINT ( 'NONE',  ( 69.52686081652188932, 40.65493879156205281, 28.12500000000001066 ) ) ;
#6510=CARTESIAN_POINT ( 'NONE',  ( 76.84714931290172046, 44.87559967700520502, 21.12007276954038915 ) ) ;
#6519=ORIENTED_EDGE ( 'NONE', *, *, #6608, .T. ) ;
#6527=LINE ( 'NONE', #11622, #500 ) ;
#6528=CARTESIAN_POINT ( 'NONE',  ( -8.022189948025989281, 43.39365864146846263, 74.57502254044544543 ) ) ;
#6531=CARTESIAN_POINT ( 'NONE',  ( 7.007733291640687590, 17.40453028225516974, 74.67565132020823171 ) ) ;
#6533=AXIS2_PLACEMENT_3D ( 'NONE', #370, #252, #3242 ) ;
#6536=DIRECTION ( 'NONE',  ( 0.000000000000000000, 0.000000000000000000, -1.000000000000000000 ) ) ;
#6541=ORIENTED_EDGE ( 'NONE', *, *, #5783, .F. ) ;
#6543=AXIS2_PLACEMENT_3D ( 'NONE', #11005, #2468, #10060 ) ;
#6547=ORIENTED_EDGE ( 'NONE', *, *, #4136, .F. ) ;
#6549=ORIENTED_EDGE ( 'NONE', *, *, #9770, .T. ) ;
#6551=EDGE_CURVE ( 'NONE', #2768, #1231, #1846, .T. ) ;
#6555=VERTEX_POINT ( 'NONE', #4239 ) ;
#6557=VECTOR ( 'NONE', #2031, 1000.000000000000000 ) ;
#6558=EDGE_CURVE ( 'NONE', #5372, #10740, #9906, .T. ) ;
#6559=EDGE_LOOP ( 'NONE', ( #1144, #6170, #4035, #3338 ) ) ;
#6561=CARTESIAN_POINT ( 'NONE',  ( -14.50972348255446320, 23.02286878654513202, 73.58429599720173542 ) ) ;
#6565=ORIENTED_EDGE ( 'NONE', *, *, #9080, .F. ) ;
#6570=DIRECTION ( 'NONE',  ( -3.469446951953613203E-16, 0.000000000000000000, -1.000000000000000000 ) ) ;
#6573=EDGE_CURVE ( 'NONE', #8283, #8585, #2845, .T. ) ;
#6577=DIRECTION ( 'NONE',  ( 0.000000000000000000, 0.000000000000000000, -1.000000000000000000 ) ) ;
#6581=CARTESIAN_POINT ( 'NONE',  ( -14.01037901404159669, 37.85720668004749712, 73.68231848073395440 ) ) ;
#6584=AXIS2_PLACEMENT_3D ( 'NONE', #4633, #963, #9358 ) ;
#6585=AXIS2_PLACEMENT_3D ( 'NONE', #10378, #1666, #5658 ) ;
#6587=CARTESIAN_POINT ( 'NONE',  ( 70.87894850892848808, 41.68318366108226058, -24.74065748999147019 ) ) ;
#6588=CARTESIAN_POINT ( 'NONE',  ( 75.00000000000001421, 15.00000000000008882, 20.00000000000000000 ) ) ;
#6591=TOROIDAL_SURFACE ( 'NONE', #5604, 25.00000000000000000, 10.00000000000000000 ) ;
#6595=ORIENTED_EDGE ( 'NONE', *, *, #6127, .T. ) ;
#6603=ORIENTED_EDGE ( 'NONE', *, *, #3487, .T. ) ;
#6604=ADVANCED_FACE ( 'NONE', ( #5185 ), #11101, .T. ) ;
#6608=EDGE_CURVE ( 'NONE', #7410, #2768, #8803, .T. ) ;
#6614=DIRECTION ( 'NONE',  ( 6.938893903907221475E-16, 0.000000000000000000, -1.000000000000000000 ) ) ;
#6618=AXIS2_PLACEMENT_3D ( 'NONE', #4582, #9183, #10119 ) ;
#6619=VERTEX_POINT ( 'NONE', #437 ) ;
#6622=CARTESIAN_POINT ( 'NONE',  ( 70.48329812536721306, 46.79482878816214253, 25.63505613512332459 ) ) ;
#6625=CARTESIAN_POINT ( 'NONE',  ( 77.29209776116496755, 45.00000000000009237, 20.32449628861576940 ) ) ;
#6641=DIRECTION ( 'NONE',  ( 0.000000000000000000, 1.000000000000000000, 0.000000000000000000 ) ) ;
#6644=DIRECTION ( 'NONE',  ( -0.000000000000000000, 1.000000000000000000, -0.000000000000000000 ) ) ;
#6648=CARTESIAN_POINT ( 'NONE',  ( 69.65391855624119444, 42.66023882883560248, -27.80917345409739383 ) ) ;
#6650=EDGE_LOOP ( 'NONE', ( #12069, #6547, #3960, #4039 ) ) ;
#6652=AXIS2_PLACEMENT_3D ( 'NONE', #5326, #4510, #10926 ) ;
#6655=FACE_OUTER_BOUND ( 'NONE', #5557, .T. ) ;
#6658=EDGE_CURVE ( 'NONE', #6384, #10790, #10334, .T. ) ;
#6661=CARTESIAN_POINT ( 'NONE',  ( 165.0000000000011369, 0.000000000000000000, 20.00000000000000000 ) ) ;
#6667=CARTESIAN_POINT ( 'NONE',  ( 121.4644660940682428, 46.46446609406732620, 25.00000000000000000 ) ) ;
#6670=CARTESIAN_POINT ( 'NONE',  ( 0.000000000000000000, -5.000000000000000000, -65.00000000000001421 ) ) ;
#6674=LINE ( 'NONE', #7731, #5621 ) ;
#6683=CIRCLE ( 'NONE', #3893, 70.00000000000000000 ) ;
#6684=ORIENTED_EDGE ( 'NONE', *, *, #1029, .F. ) ;
#6686=PLANE ( 'NONE',  #2493 ) ;
#6689=FACE_OUTER_BOUND ( 'NONE', #8966, .T. ) ;
#6690=CARTESIAN_POINT ( 'NONE',  ( 70.01409082250445692, 15.02759043508419623, 26.88960057466318077 ) ) ;
#6694=AXIS2_PLACEMENT_3D ( 'NONE', #4183, #6243, #7174 ) ;
#6695=DIRECTION ( 'NONE',  ( -1.000000000000000000, 0.000000000000000000, 0.000000000000000000 ) ) ;
#6697=EDGE_CURVE ( 'NONE', #7931, #5487, #2675, .T. ) ;
#6702=CARTESIAN_POINT ( 'NONE',  ( 41.03553390593253170, -41.03553390593296513, 20.00000000000000000 ) ) ;
#6713=CARTESIAN_POINT ( 'NONE',  ( 70.79098555864042908, 40.00000000000007816, -25.00000000000000000 ) ) ;
#6714=B_SPLINE_CURVE_WITH_KNOTS ( 'NONE', 3,
 ( #11476, #2928, #10525, #1184, #1991, #4986, #5799, #1057, #3928, #2989, #7723, #10589, #5859, #9642, #4926, #10075, #6106, #6224 ),
 .UNSPECIFIED., .F., .F.,
 ( 4, 2, 2, 2, 2, 2, 2, 2, 4 ),
 ( 0.000000000000000000, 0.001070893387785250587, 0.002141786775570501174, 0.003212680163355751545, 0.004283573551141002349, 0.005354466938926253153, 0.006425360326711503089, 0.007496253714496753894, 0.008567147102282004698 ),
 .UNSPECIFIED. ) ;
#6717=CARTESIAN_POINT ( 'NONE',  ( 9.184850993605150311E-15, 50.00000000000000000, 75.00000000000001421 ) ) ;
#6731=LINE ( 'NONE', #5924, #924 ) ;
#6733=ADVANCED_FACE ( 'NONE', ( #2737 ), #11349, .F. ) ;
#6747=DIRECTION ( 'NONE',  ( 0.000000000000000000, 0.000000000000000000, 1.000000000000000000 ) ) ;
#6757=VERTEX_POINT ( 'NONE', #9395 ) ;
#6758=CARTESIAN_POINT ( 'NONE',  ( 9.514435292357342533, 40.51730218646115844, 74.39473334479674804 ) ) ;
#6768=AXIS2_PLACEMENT_3D ( 'NONE', #5889, #9670, #382 ) ;
#6772=CARTESIAN_POINT ( 'NONE',  ( 71.69656859387023928, 44.65045859775734982, -22.14271594285822431 ) ) ;
#6773=EDGE_CURVE ( 'NONE', #10965, #5376, #858, .T. ) ;
#6775=PLANE ( 'NONE',  #1027 ) ;
#6777=CARTESIAN_POINT ( 'NONE',  ( 71.54748821555645577, 15.63447443924222569, -22.64388168111003807 ) ) ;
#6785=EDGE_CURVE ( 'NONE', #357, #10533, #9518, .T. ) ;
#6786=( BOUNDED_CURVE ( )  B_SPLINE_CURVE ( 3, ( #10683, #9735, #270, #5832 ),
 .UNSPECIFIED., .F., .F. ) 
 B_SPLINE_CURVE_WITH_KNOTS ( ( 4, 4 ),
 ( 0.000000000000000000, 1.570796326794896558 ),
 .UNSPECIFIED. ) 
 CURVE ( )  GEOMETRIC_REPRESENTATION_ITEM ( )  RATIONAL_B_SPLINE_CURVE ( ( 1.000000000000000000, 0.8047378541243649375, 0.8047378541243649375, 1.000000000000000000 ) ) 
 REPRESENTATION_ITEM ( '' )  );
#6787=VECTOR ( 'NONE', #4028, 1000.000000000000000 ) ;
#6792=DIRECTION ( 'NONE',  ( -0.7071067811865513475, -0.7071067811865437980, -0.000000000000000000 ) ) ;
#6819=ADVANCED_FACE ( 'NONE', ( #5982 ), #7897, .F. ) ;
#6824=CARTESIAN_POINT ( 'NONE',  ( 0.9349062160761316687, 44.87820708871510789, 75.00000000000002842 ) ) ;
#6830=DIRECTION ( 'NONE',  ( 0.000000000000000000, 0.000000000000000000, 1.000000000000000000 ) ) ;
#6831=ORIENTED_EDGE ( 'NONE', *, *, #10610, .T. ) ;
#6833=( NAMED_UNIT ( * ) PLANE_ANGLE_UNIT ( ) SI_UNIT ( $, .RADIAN. ) );
#6836=EDGE_CURVE ( 'NONE', #10533, #8585, #3986, .T. ) ;
#6842=CARTESIAN_POINT ( 'NONE',  ( 71.59683363033870762, 15.53272889911889543, -22.47949853503603990 ) ) ;
#6851=CIRCLE ( 'NONE', #12237, 5.000000000000004441 ) ;
#6857=LINE ( 'NONE', #9587, #11277 ) ;
#6859=SHAPE_DEFINITION_REPRESENTATION ( #3790, #9674 ) ;
#6869=CARTESIAN_POINT ( 'NONE',  ( 0.000000000000000000, 115.0000000000000000, 0.000000000000000000 ) ) ;
#6871=EDGE_LOOP ( 'NONE', ( #8229, #7361, #5353, #515, #10912, #4593, #1989, #121 ) ) ;
#6873=DIRECTION ( 'NONE',  ( 0.000000000000000000, 1.000000000000000000, 0.000000000000000000 ) ) ;
#6890=ORIENTED_EDGE ( 'NONE', *, *, #4636, .T. ) ;
#6897=EDGE_CURVE ( 'NONE', #9831, #4212, #6714, .T. ) ;
#6901=CIRCLE ( 'NONE', #7883, 10.00000000000000178 ) ;
#6907=CARTESIAN_POINT ( 'NONE',  ( 74.98782882127120786, 16.91249280870930605, -23.93624459205407362 ) ) ;
#6912=VECTOR ( 'NONE', #10548, 1000.000000000000000 ) ;
#6919=ORIENTED_EDGE ( 'NONE', *, *, #3661, .T. ) ;
#6922=CARTESIAN_POINT ( 'NONE',  ( 30.00000000000004263, 65.00000000000000000, -63.24555320336758513 ) ) ;
#6929=DIRECTION ( 'NONE',  ( 1.000000000000000000, -0.000000000000000000, 0.000000000000000000 ) ) ;
#6931=ORIENTED_EDGE ( 'NONE', *, *, #1333, .T. ) ;
#6933=CARTESIAN_POINT ( 'NONE',  ( 69.64721689463594601, 17.41064966062540620, 27.82591776719579713 ) ) ;
#6943=AXIS2_PLACEMENT_3D ( 'NONE', #9489, #2588, #6577 ) ;
#6945=CARTESIAN_POINT ( 'NONE',  ( 77.29025109341738187, 45.00000000000009237, -20.32807234521402151 ) ) ;
#6948=CARTESIAN_POINT ( 'NONE',  ( 8.485645551905516726, 41.47111475299955430, 74.51923978935600701 ) ) ;
#6951=DIRECTION ( 'NONE',  ( 0.000000000000000000, 0.000000000000000000, -1.000000000000000000 ) ) ;
#6954=EDGE_LOOP ( 'NONE', ( #11066, #6890, #9687, #8176, #2821, #9616, #5432, #4540, #4485 ) ) ;
#6960=FACE_OUTER_BOUND ( 'NONE', #4975, .T. ) ;
#6987=LINE ( 'NONE', #9718, #5081 ) ;
#6994=DIRECTION ( 'NONE',  ( -0.000000000000000000, 1.000000000000000000, -0.000000000000000000 ) ) ;
#6997=DIRECTION ( 'NONE',  ( 1.000000000000000000, 0.000000000000000000, 0.000000000000000000 ) ) ;
#6999=CARTESIAN_POINT ( 'NONE',  ( 72.13972991038781402, 14.87494484084908386, 20.57104709750045402 ) ) ;
#7003=CARTESIAN_POINT ( 'NONE',  ( 74.62554477486000337, 17.62767568092783321, 24.41456952963950755 ) ) ;
#7004=CARTESIAN_POINT ( 'NONE',  ( 76.19556706709904859, 44.50529433006728652, -22.19251267860074961 ) ) ;
#7005=EDGE_LOOP ( 'NONE', ( #9464, #2308, #9711, #5355 ) ) ;
#7009=CARTESIAN_POINT ( 'NONE',  ( 70.79098555864042908, 40.00000000000009237, 25.00000000000000000 ) ) ;
#7015=EDGE_CURVE ( 'NONE', #8096, #11474, #3361, .T. ) ;
#7017=ORIENTED_EDGE ( 'NONE', *, *, #4354, .T. ) ;
#7019=CIRCLE ( 'NONE', #10194, 5.000000000000001776 ) ;
#7037=CARTESIAN_POINT ( 'NONE',  ( -20.00000000000000355, 7.965803112215716020, -57.08203932499370836 ) ) ;
#7041=ORIENTED_EDGE ( 'NONE', *, *, #10028, .F. ) ;
#7042=CARTESIAN_POINT ( 'NONE',  ( 69.85318522031718658, 44.10340835627246037, -27.30472166927799194 ) ) ;
#7048=DIRECTION ( 'NONE',  ( 0.000000000000000000, 0.000000000000000000, 1.000000000000000000 ) ) ;
#7053=ORIENTED_EDGE ( 'NONE', *, *, #11746, .F. ) ;
#7057=CARTESIAN_POINT ( 'NONE',  ( 20.00000000000000711, 63.00000000000000000, 67.08203932499370126 ) ) ;
#7058=DIRECTION ( 'NONE',  ( -1.000000000000000000, -0.000000000000000000, 0.000000000000000000 ) ) ;
#7061=CARTESIAN_POINT ( 'NONE',  ( 76.01088325117457600, 15.64455795939924698, 22.47665947743448100 ) ) ;
#7065=CARTESIAN_POINT ( 'NONE',  ( 72.32495769890020654, 45.16153383718148007, -19.87825060515872266 ) ) ;
#7069=CARTESIAN_POINT ( 'NONE',  ( 70.96239324365633649, 42.26132884148638880, 24.49110472308180064 ) ) ;
#7076=CIRCLE ( 'NONE', #2499, 5.000000000000000888 ) ;
#7085=DIRECTION ( 'NONE',  ( 0.000000000000000000, 0.000000000000000000, 1.000000000000000000 ) ) ;
#7091=CARTESIAN_POINT ( 'NONE',  ( 72.61843774138908714, 10.00000000000017586, -18.75000000000000000 ) ) ;
#7100=CARTESIAN_POINT ( 'NONE',  ( 76.23530124607876246, 15.46574672446569387, -22.12995508525856536 ) ) ;
#7114=DIRECTION ( 'NONE',  ( 0.000000000000000000, 0.000000000000000000, 1.000000000000000000 ) ) ;
#7118=CYLINDRICAL_SURFACE ( 'NONE', #9877, 5.000000000000001776 ) ;
#7122=CARTESIAN_POINT ( 'NONE',  ( 76.75412411316109740, 15.16378490115497080, 21.27950340534427198 ) ) ;
#7125=CARTESIAN_POINT ( 'NONE',  ( 77.11525298301567943, 44.96802867796342440, -20.64974928742854132 ) ) ;
#7127=ORIENTED_EDGE ( 'NONE', *, *, #5014, .T. ) ;
#7129=CARTESIAN_POINT ( 'NONE',  ( 74.26978800665389713, 41.16139233038059331, 24.86610009102963659 ) ) ;
#7146=CARTESIAN_POINT ( 'NONE',  ( 120.0000000000009948, 45.00000000000008527, 20.00000000000000000 ) ) ;
#7148=CARTESIAN_POINT ( 'NONE',  ( 74.16198487095665826, 40.00000000000009237, 25.00000000000000000 ) ) ;
#7151=FACE_OUTER_BOUND ( 'NONE', #462, .T. ) ;
#7156=CARTESIAN_POINT ( 'NONE',  ( 170.0000000000011369, 230.0000000000000853, -19.99999999999999645 ) ) ;
#7159=CARTESIAN_POINT ( 'NONE',  ( 125.0000000000009663, 42.92893218813457423, 25.00000000000000000 ) ) ;
#7163=DIRECTION ( 'NONE',  ( 1.000000000000000000, -0.000000000000000000, -0.000000000000000000 ) ) ;
#7165=CARTESIAN_POINT ( 'NONE',  ( 147.9289321881356045, 20.00000000000009237, 25.00000000000000000 ) ) ;
#7169=EDGE_LOOP ( 'NONE', ( #682, #7297, #11160, #7754 ) ) ;
#7174=DIRECTION ( 'NONE',  ( 0.000000000000000000, -0.000000000000000000, 1.000000000000000000 ) ) ;
#7178=CARTESIAN_POINT ( 'NONE',  ( 69.52686081652184669, 40.00000000000009237, -28.12499999999999645 ) ) ;
#7180=AXIS2_PLACEMENT_3D ( 'NONE', #8197, #353, #9125 ) ;
#7181=ORIENTED_EDGE ( 'NONE', *, *, #9998, .F. ) ;
#7185=CARTESIAN_POINT ( 'NONE',  ( 70.82643617010576520, 18.93883522538484243, 24.89585111362008263 ) ) ;
#7191=CARTESIAN_POINT ( 'NONE',  ( 71.69660397288474485, 44.65047563280165122, 22.14258685050887010 ) ) ;
#7193=FACE_OUTER_BOUND ( 'NONE', #2929, .T. ) ;
#7198=ORIENTED_EDGE ( 'NONE', *, *, #3119, .T. ) ;
#7206=CARTESIAN_POINT ( 'NONE',  ( 140.0000000000011369, 225.0000000000000853, 25.00000000000000000 ) ) ;
#7212=CARTESIAN_POINT ( 'NONE',  ( 69.72092797052474111, 16.81038406663796536, -27.64057077031494458 ) ) ;
#7218=AXIS2_PLACEMENT_3D ( 'NONE', #5836, #6641, #2090 ) ;
#7223=CARTESIAN_POINT ( 'NONE',  ( 0.000000000000000000, 10.00000000000017586, 0.000000000000000000 ) ) ;
#7226=DIRECTION ( 'NONE',  ( -0.000000000000000000, 0.000000000000000000, 1.000000000000000000 ) ) ;
#7239=CARTESIAN_POINT ( 'NONE',  ( 72.02465572632023338, 10.26536114380532894, 20.91766802171319739 ) ) ;
#7243=CARTESIAN_POINT ( 'NONE',  ( 0.000000000000000000, 75.00000000000000000, 0.000000000000000000 ) ) ;
#7249=CARTESIAN_POINT ( 'NONE',  ( 71.06140945339295456, 17.19704224702771356, 24.19089746873543945 ) ) ;
#7257=FACE_OUTER_BOUND ( 'NONE', #6559, .T. ) ;
#7258=CARTESIAN_POINT ( 'NONE',  ( 69.62792625627750454, 42.32278466075560175, 27.87393767067159089 ) ) ;
#7264=VECTOR ( 'NONE', #7989, 1000.000000000000000 ) ;
#7277=DIRECTION ( 'NONE',  ( -0.000000000000000000, -1.000000000000000000, -0.000000000000000000 ) ) ;
#7283=CARTESIAN_POINT ( 'NONE',  ( 13.80921887069452758, 30.00000000000009237, 73.71774192269630532 ) ) ;
#7291=AXIS2_PLACEMENT_3D ( 'NONE', #10910, #10851, #5188 ) ;
#7293=DIRECTION ( 'NONE',  ( 0.000000000000000000, 0.000000000000000000, 1.000000000000000000 ) ) ;
#7297=ORIENTED_EDGE ( 'NONE', *, *, #2585, .T. ) ;
#7298=ORIENTED_EDGE ( 'NONE', *, *, #6551, .F. ) ;
#7300=DIRECTION ( 'NONE',  ( 0.000000000000000000, 0.000000000000000000, 1.000000000000000000 ) ) ;
#7303=VECTOR ( 'NONE', #6994, 1000.000000000000000 ) ;
#7304=FACE_OUTER_BOUND ( 'NONE', #11874, .T. ) ;
#7311=ORIENTED_EDGE ( 'NONE', *, *, #7715, .F. ) ;
#7322=CARTESIAN_POINT ( 'NONE',  ( 76.75496552995652166, 44.83661607564270213, 21.27808286176542296 ) ) ;
#7333=LINE ( 'NONE', #8376, #7614 ) ;
#7336=CARTESIAN_POINT ( 'NONE',  ( -9.345585736091447160, 42.60014767327400165, 74.41678175564237563 ) ) ;
#7337=VECTOR ( 'NONE', #2736, 999.9999999999998863 ) ;
#7338=CARTESIAN_POINT ( 'NONE',  ( 12.41838735530818738, 23.67465209942693960, 73.96505410671836955 ) ) ;
#7342=EDGE_CURVE ( 'NONE', #5348, #2246, #5220, .T. ) ;
#7349=CARTESIAN_POINT ( 'NONE',  ( 74.16198487146469631, 19.66102550257836512, -24.99999999999999645 ) ) ;
#7352=EDGE_CURVE ( 'NONE', #8585, #10899, #10815, .T. ) ;
#7361=ORIENTED_EDGE ( 'NONE', *, *, #6658, .F. ) ;
#7368=DIRECTION ( 'NONE',  ( -1.000000000000000000, 0.000000000000000000, -0.000000000000000000 ) ) ;
#7374=CYLINDRICAL_SURFACE ( 'NONE', #2189, 5.000000000000004441 ) ;
#7376=EDGE_CURVE ( 'NONE', #10768, #6205, #3345, .T. ) ;
#7385=CIRCLE ( 'NONE', #7180, 5.000000000000000888 ) ;
#7388=CYLINDRICAL_SURFACE ( 'NONE', #9963, 5.000000000000004441 ) ;
#7392=CIRCLE ( 'NONE', #6584, 70.00000000000001421 ) ;
#7396=AXIS2_PLACEMENT_3D ( 'NONE', #1976, #5786, #4915 ) ;
#7397=DIRECTION ( 'NONE',  ( 1.000000000000000000, -0.000000000000000000, 0.000000000000000000 ) ) ;
#7401=CARTESIAN_POINT ( 'NONE',  ( -15.31738143124597151, 35.07030106808286263, 73.41937046907847275 ) ) ;
#7403=EDGE_CURVE ( 'NONE', #9072, #8789, #8129, .T. ) ;
#7404=EDGE_CURVE ( 'NONE', #3822, #5087, #1860, .T. ) ;
#7409=CARTESIAN_POINT ( 'NONE',  ( 1.088204915335219061E-15, 15.04734002586538821, 75.00000000000001421 ) ) ;
#7410=VERTEX_POINT ( 'NONE', #5279 ) ;
#7413=CARTESIAN_POINT ( 'NONE',  ( 70.86094439463602157, 18.52957660828512587, -24.79386831724005091 ) ) ;
#7422=AXIS2_PLACEMENT_3D ( 'NONE', #273, #11695, #5956 ) ;
#7423=DIRECTION ( 'NONE',  ( -0.000000000000000000, -1.000000000000000000, -0.000000000000000000 ) ) ;
#7430=EDGE_CURVE ( 'NONE', #7410, #11037, #10421, .T. ) ;
#7434=EDGE_LOOP ( 'NONE', ( #6549, #2230, #6684, #8774 ) ) ;
#7440=CARTESIAN_POINT ( 'NONE',  ( -16.16361926974168384, 28.95936500225007748, 73.23756171298010997 ) ) ;
#7443=CARTESIAN_POINT ( 'NONE',  ( 72.28042146286416880, 45.16208194665043862, 20.04664579644909139 ) ) ;
#7447=PLANE ( 'NONE',  #2012 ) ;
#7455=CARTESIAN_POINT ( 'NONE',  ( 3.061616997868383043E-15, 65.00000000000000000, -25.00000000000000000 ) ) ;
#7468=CARTESIAN_POINT ( 'NONE',  ( 6.215335591258955183, 16.92236976696375805, 74.74677668485156801 ) ) ;
#7469=VECTOR ( 'NONE', #7854, 1000.000000000000000 ) ;
#7479=CARTESIAN_POINT ( 'NONE',  ( -20.00000000000000355, 50.00000000000000000, 57.08203932499370836 ) ) ;
#7485=CIRCLE ( 'NONE', #7291, 75.00000000000001421 ) ;
#7495=EDGE_CURVE ( 'NONE', #11350, #3728, #3236, .T. ) ;
#7500=CARTESIAN_POINT ( 'NONE',  ( 70.63701798748766691, 47.25584164860985226, 25.20839359252511969 ) ) ;
#7501=ORIENTED_EDGE ( 'NONE', *, *, #8805, .T. ) ;
#7503=CARTESIAN_POINT ( 'NONE',  ( 0.000000000000000000, 50.00000000000000000, 0.000000000000000000 ) ) ;
#7511=DIRECTION ( 'NONE',  ( 0.7071067811865513475, 0.7071067811865437980, 0.000000000000000000 ) ) ;
#7515=CARTESIAN_POINT ( 'NONE',  ( 0.000000000000000000, 50.00000000000000000, 0.000000000000000000 ) ) ;
#7516=( BOUNDED_CURVE ( )  B_SPLINE_CURVE ( 3, ( #3346, #7944, #3279, #11771 ),
 .UNSPECIFIED., .F., .F. ) 
 B_SPLINE_CURVE_WITH_KNOTS ( ( 4, 4 ),
 ( 1.860548028230944562, 2.013707370868536461 ),
 .UNSPECIFIED. ) 
 CURVE ( )  GEOMETRIC_REPRESENTATION_ITEM ( )  RATIONAL_B_SPLINE_CURVE ( ( 1.000000000000000000, 0.9980461397859388128, 0.9980461397859388128, 1.000000000000000000 ) ) 
 REPRESENTATION_ITEM ( '' )  );
#7519=LINE ( 'NONE', #5595, #5194 ) ;
#7523=DIRECTION ( 'NONE',  ( 0.000000000000000000, 0.7071067811865514585, 0.7071067811865435759 ) ) ;
#7524=LINE ( 'NONE', #6588, #8263 ) ;
#7528=DIRECTION ( 'NONE',  ( -0.000000000000000000, -1.000000000000000000, -0.000000000000000000 ) ) ;
#7529=CARTESIAN_POINT ( 'NONE',  ( 74.26978800665389713, 18.83860766962025224, -24.86610009102977159 ) ) ;
#7530=EDGE_LOOP ( 'NONE', ( #2584, #6420, #10560, #5526 ) ) ;
#7533=ORIENTED_EDGE ( 'NONE', *, *, #5111, .F. ) ;
#7539=ORIENTED_EDGE ( 'NONE', *, *, #2181, .T. ) ;
#7548=EDGE_CURVE ( 'NONE', #9474, #9178, #3531, .T. ) ;
#7549=EDGE_CURVE ( 'NONE', #9708, #11877, #7333, .T. ) ;
#7566=TOROIDAL_SURFACE ( 'NONE', #10751, 10.00000000000000000, 5.000000000000000000 ) ;
#7567=CARTESIAN_POINT ( 'NONE',  ( 0.000000000000000000, 63.00000000000000000, -57.08203932499371547 ) ) ;
#7568=EDGE_LOOP ( 'NONE', ( #3618, #3832, #12304, #7594, #2299, #628, #4619, #2731, #4165, #7198 ) ) ;
#7571=CARTESIAN_POINT ( 'NONE',  ( -20.00000000000000355, 7.965803112215716020, -57.08203932499370836 ) ) ;
#7576=LINE ( 'NONE', #1035, #6557 ) ;
#7581=CARTESIAN_POINT ( 'NONE',  ( 74.16198487095664404, 40.00000000000008527, -25.00000000000000000 ) ) ;
#7585=EDGE_CURVE ( 'NONE', #737, #8283, #8598, .T. ) ;
#7587=CARTESIAN_POINT ( 'NONE',  ( 8.266365894244636700E-15, -10.00000000000000000, 65.00000000000001421 ) ) ;
#7588=CARTESIAN_POINT ( 'NONE',  ( 69.77609205918946600, 16.39783078570843244, -27.50116345873387758 ) ) ;
#7594=ORIENTED_EDGE ( 'NONE', *, *, #7549, .T. ) ;
#7607=CARTESIAN_POINT ( 'NONE',  ( 165.0000000000011369, 225.0000000000000853, 25.00000000000000000 ) ) ;
#7614=VECTOR ( 'NONE', #7397, 1000.000000000000000 ) ;
#7618=CARTESIAN_POINT ( 'NONE',  ( 70.00771527461461119, 44.96961139197239277, 26.90815449096327683 ) ) ;
#7621=CARTESIAN_POINT ( 'NONE',  ( 69.53296405455486706, 19.34582284458782553, 28.10992626845828113 ) ) ;
#7624=CARTESIAN_POINT ( 'NONE',  ( 135.0000000000011084, 67.07106781186550393, 25.00000000000000000 ) ) ;
#7633=CARTESIAN_POINT ( 'NONE',  ( 9.182979779718706936, 40.84457429296963227, 74.43652437870400718 ) ) ;
#7645=CARTESIAN_POINT ( 'NONE',  ( 70.82643617010577941, 41.06116477461475966, -24.89585111361949643 ) ) ;
#7646=( NAMED_UNIT ( * ) PLANE_ANGLE_UNIT ( ) SI_UNIT ( $, .RADIAN. ) );
#7648=AXIS2_PLACEMENT_3D ( 'NONE', #5575, #1016, #3883 ) ;
#7649=CARTESIAN_POINT ( 'NONE',  ( 140.0000000000011369, 225.0000000000000853, -20.00000000000000000 ) ) ;
#7651=CARTESIAN_POINT ( 'NONE',  ( 71.74731260882261097, 15.26788291291094168, -21.96902955818390168 ) ) ;
#7652=ORIENTED_EDGE ( 'NONE', *, *, #6127, .F. ) ;
#7655=ORIENTED_EDGE ( 'NONE', *, *, #11767, .F. ) ;
#7667=VECTOR ( 'NONE', #1382, 1000.000000000000000 ) ;
#7673=EDGE_CURVE ( 'NONE', #7980, #8527, #11810, .T. ) ;
#7675=ORIENTED_EDGE ( 'NONE', *, *, #7715, .T. ) ;
#7677=CARTESIAN_POINT ( 'NONE',  ( -7.076627832483614711, 16.19342887763680494, 74.66686486294869951 ) ) ;
#7679=VERTEX_POINT ( 'NONE', #5652 ) ;
#7681=CARTESIAN_POINT ( 'NONE',  ( 138.5355339059338462, 63.53553390593273775, 20.00000000000000000 ) ) ;
#7686=AXIS2_PLACEMENT_3D ( 'NONE', #6430, #5434, #8221 ) ;
#7690=CARTESIAN_POINT ( 'NONE',  ( 72.45961080413260902, 10.00000000123442412, 19.36513408292344351 ) ) ;
#7700=AXIS2_PLACEMENT_3D ( 'NONE', #8672, #4690, #5702 ) ;
#7705=ADVANCED_FACE ( 'NONE', ( #4960 ), #2030, .T. ) ;
#7708=CARTESIAN_POINT ( 'NONE',  ( 75.47338808840343916, 43.79030468642783092, -23.26499062814251317 ) ) ;
#7709=SURFACE_STYLE_FILL_AREA ( #3780 ) ;
#7711=DIRECTION ( 'NONE',  ( 0.000000000000000000, 1.000000000000000000, 0.000000000000000000 ) ) ;
#7712=CARTESIAN_POINT ( 'NONE',  ( 20.00000000000000355, 7.965803112215716020, -57.08203932499370836 ) ) ;
#7713=CARTESIAN_POINT ( 'NONE',  ( 75.47443053502085775, 16.20845120114963933, -23.26350036030322954 ) ) ;
#7715=EDGE_CURVE ( 'NONE', #357, #11448, #7019, .T. ) ;
#7723=CARTESIAN_POINT ( 'NONE',  ( 75.70364277637114014, 44.05991784979070047, 22.93512150616605538 ) ) ;
#7731=CARTESIAN_POINT ( 'NONE',  ( 20.00000000000000711, 63.00000000000000000, 67.08203932499370126 ) ) ;
#7733=AXIS2_PLACEMENT_3D ( 'NONE', #5128, #8904, #6175 ) ;
#7739=VERTEX_POINT ( 'NONE', #11571 ) ;
#7742=ORIENTED_EDGE ( 'NONE', *, *, #3831, .T. ) ;
#7746=EDGE_CURVE ( 'NONE', #9696, #3575, #9429, .T. ) ;
#7750=CARTESIAN_POINT ( 'NONE',  ( 72.61843774138908714, 10.00000000000009059, 18.75000000000000355 ) ) ;
#7752=ORIENTED_EDGE ( 'NONE', *, *, #1892, .F. ) ;
#7754=ORIENTED_EDGE ( 'NONE', *, *, #8075, .F. ) ;
#7755=CARTESIAN_POINT ( 'NONE',  ( 147.9289321881356045, 20.00000000000008527, -25.00000000000000000 ) ) ;
#7757=ORIENTED_EDGE ( 'NONE', *, *, #7430, .F. ) ;
#7761=DIRECTION ( 'NONE',  ( 0.000000000000000000, 0.000000000000000000, 1.000000000000000000 ) ) ;
#7771=CARTESIAN_POINT ( 'NONE',  ( 70.92186449036606177, 12.01005621119159450, -24.39573567383822095 ) ) ;
#7775=FACE_OUTER_BOUND ( 'NONE', #571, .T. ) ;
#7778=VECTOR ( 'NONE', #9619, 1000.000000000000000 ) ;
#7783=DIRECTION ( 'NONE',  ( -0.000000000000000000, -0.000000000000000000, 1.000000000000000000 ) ) ;
#7793=EDGE_LOOP ( 'NONE', ( #9334, #1407, #3851, #10681 ) ) ;
#7794=CARTESIAN_POINT ( 'NONE',  ( 150.0000000000010800, 15.00000000000008882, 20.00000000000000000 ) ) ;
#7796=EDGE_CURVE ( 'NONE', #4313, #4047, #11208, .T. ) ;
#7798=VECTOR ( 'NONE', #4152, 1000.000000000000000 ) ;
#7801=CARTESIAN_POINT ( 'NONE',  ( 145.0000000000011369, 225.0000000000000853, -20.00000000000000000 ) ) ;
#7803=CARTESIAN_POINT ( 'NONE',  ( 1.088204915335219061E-15, 15.04734002586538821, 75.00000000000001421 ) ) ;
#7805=DIRECTION ( 'NONE',  ( -1.000000000000000000, 0.000000000000000000, 0.000000000000000000 ) ) ;
#7806=CARTESIAN_POINT ( 'NONE',  ( 69.55717041450677129, 18.69586594910642319, 28.04997484771492466 ) ) ;
#7809=LINE ( 'NONE', #11623, #6912 ) ;
#7812=DIRECTION ( 'NONE',  ( -0.000000000000000000, -1.000000000000000000, -0.000000000000000000 ) ) ;
#7818=CARTESIAN_POINT ( 'NONE',  ( 1.850901974874337830, 44.71779529743732695, 74.98253729624308050 ) ) ;
#7819=ORIENTED_EDGE ( 'NONE', *, *, #3331, .T. ) ;
#7823=DIRECTION ( 'NONE',  ( 0.000000000000000000, 0.000000000000000000, 1.000000000000000000 ) ) ;
#7825=VECTOR ( 'NONE', #2417, 1000.000000000000000 ) ;
#7831=CARTESIAN_POINT ( 'NONE',  ( 77.11786746747833377, 15.03129260902921516, -20.64504863446460803 ) ) ;
#7838=TOROIDAL_SURFACE ( 'NONE', #9219, 10.00000000000000000, 5.000000000000000000 ) ;
#7839=VERTEX_POINT ( 'NONE', #335 ) ;
#7841=CARTESIAN_POINT ( 'NONE',  ( 120.0000000000010090, 45.00000000000009237, -20.00000000000000000 ) ) ;
#7842=ORIENTED_EDGE ( 'NONE', *, *, #10645, .F. ) ;
#7854=DIRECTION ( 'NONE',  ( -0.000000000000000000, -0.000000000000000000, 1.000000000000000000 ) ) ;
#7870=ORIENTED_EDGE ( 'NONE', *, *, #9304, .T. ) ;
#7871=ORIENTED_EDGE ( 'NONE', *, *, #4668, .F. ) ;
#7874=CARTESIAN_POINT ( 'NONE',  ( 11.02221580535522172, 38.75872166009053643, 74.18734971499729625 ) ) ;
#7880=DIRECTION ( 'NONE',  ( 2.213536252433181319E-16, 0.000000000000000000, 1.000000000000000000 ) ) ;
#7881=TOROIDAL_SURFACE ( 'NONE', #10860, 65.00000000000001421, 5.000000000000000000 ) ;
#7883=AXIS2_PLACEMENT_3D ( 'NONE', #12083, #6401, #10188 ) ;
#7888=CARTESIAN_POINT ( 'NONE',  ( 72.54053945714667861, 14.91954699701732423, -19.05169875840561389 ) ) ;
#7889=DIRECTION ( 'NONE',  ( -0.000000000000000000, -1.000000000000000000, -0.000000000000000000 ) ) ;
#7895=EDGE_CURVE ( 'NONE', #6417, #9081, #4203, .T. ) ;
#7897=PLANE ( 'NONE',  #9200 ) ;
#7910=CARTESIAN_POINT ( 'NONE',  ( -10.61565724859829096, 18.28584071866657013, 74.24882261665963767 ) ) ;
#7913=CARTESIAN_POINT ( 'NONE',  ( 71.75867793008815454, 10.54280999270224406, 21.81257403104604720 ) ) ;
#7919=CARTESIAN_POINT ( 'NONE',  ( 74.19409830870891653, 40.72200583775279625, -24.96047248796921281 ) ) ;
#7922=DIRECTION ( 'NONE',  ( 0.000000000000000000, 0.000000000000000000, 1.000000000000000000 ) ) ;
#7923=CARTESIAN_POINT ( 'NONE',  ( 74.58430552652164636, 17.74813588577157475, 24.46729545492024016 ) ) ;
#7927=CARTESIAN_POINT ( 'NONE',  ( 71.89703483713221033, 44.94224125782246659, -21.44956398270095121 ) ) ;
#7929=LINE ( 'NONE', #2086, #2475 ) ;
#7930=CARTESIAN_POINT ( 'NONE',  ( 72.14031151490229377, 45.12527760491855844, 20.56889282980839440 ) ) ;
#7931=VERTEX_POINT ( 'NONE', #10747 ) ;
#7934=FACE_OUTER_BOUND ( 'NONE', #11865, .T. ) ;
#7940=VECTOR ( 'NONE', #1578, 1000.000000000000000 ) ;
#7944=CARTESIAN_POINT ( 'NONE',  ( 23.42809864819168553, 58.42809864819167132, -66.05997777686947359 ) ) ;
#7946=LINE ( 'NONE', #8941, #8476 ) ;
#7949=VECTOR ( 'NONE', #8854, 999.9999999999998863 ) ;
#7954=ORIENTED_EDGE ( 'NONE', *, *, #9074, .F. ) ;
#7957=EDGE_LOOP ( 'NONE', ( #4006, #7742, #9487, #6595 ) ) ;
#7958=FACE_OUTER_BOUND ( 'NONE', #1052, .T. ) ;
#7965=AXIS2_PLACEMENT_3D ( 'NONE', #4144, #8929, #7761 ) ;
#7968=AXIS2_PLACEMENT_3D ( 'NONE', #8907, #11495, #9602 ) ;
#7970=FACE_OUTER_BOUND ( 'NONE', #3691, .T. ) ;
#7973=CYLINDRICAL_SURFACE ( 'NONE', #5212, 5.000000000000000888 ) ;
#7978=CARTESIAN_POINT ( 'NONE',  ( 77.29385721799278031, 45.00000000000009237, -20.32108911529004303 ) ) ;
#7979=FACE_OUTER_BOUND ( 'NONE', #1864, .T. ) ;
#7980=VERTEX_POINT ( 'NONE', #3458 ) ;
#7981=DIRECTION ( 'NONE',  ( -0.000000000000000000, 1.000000000000000000, -0.000000000000000000 ) ) ;
#7983=CARTESIAN_POINT ( 'NONE',  ( 71.30804307394105024, 16.23735240717352468, 23.42323195207305986 ) ) ;
#7986=EDGE_CURVE ( 'NONE', #9490, #10391, #6385, .T. ) ;
#7987=ORIENTED_EDGE ( 'NONE', *, *, #4420, .F. ) ;
#7988=CARTESIAN_POINT ( 'NONE',  ( 75.53289395085349156, 16.12981783768338673, 23.18166983250910818 ) ) ;
#7989=DIRECTION ( 'NONE',  ( -1.000000000000000000, -0.000000000000000000, -0.000000000000000000 ) ) ;
#7992=ORIENTED_EDGE ( 'NONE', *, *, #2906, .F. ) ;
#7998=( BOUNDED_CURVE ( )  B_SPLINE_CURVE ( 3, ( #12011, #3467, #730, #8374 ),
 .UNSPECIFIED., .F., .F. ) 
 B_SPLINE_CURVE_WITH_KNOTS ( ( 4, 4 ),
 ( 4.712388980384687898, 6.283185307179586232 ),
 .UNSPECIFIED. ) 
 CURVE ( )  GEOMETRIC_REPRESENTATION_ITEM ( )  RATIONAL_B_SPLINE_CURVE ( ( 1.000000000000000000, 0.8047378541243646044, 0.8047378541243646044, 1.000000000000000000 ) ) 
 REPRESENTATION_ITEM ( '' )  );
#7999=ORIENTED_EDGE ( 'NONE', *, *, #12269, .F. ) ;
#8003=LINE ( 'NONE', #5527, #1890 ) ;
#8018=ORIENTED_EDGE ( 'NONE', *, *, #2540, .F. ) ;
#8022=CARTESIAN_POINT ( 'NONE',  ( 74.75199569173395275, 17.34624747208905760, -24.25052255086779240 ) ) ;
#8024=DIRECTION ( 'NONE',  ( 0.000000000000000000, 0.000000000000000000, -1.000000000000000000 ) ) ;
#8027=CARTESIAN_POINT ( 'NONE',  ( 70.71510656582535148, 47.48972085090039030, -24.99160257227417858 ) ) ;
#8031=PLANE ( 'NONE',  #767 ) ;
#8032=DIRECTION ( 'NONE',  ( -0.000000000000000000, 1.000000000000000000, -0.000000000000000000 ) ) ;
#8035=FACE_OUTER_BOUND ( 'NONE', #6143, .T. ) ;
#8036=EDGE_LOOP ( 'NONE', ( #890, #4751, #7311, #4680 ) ) ;
#8038=CIRCLE ( 'NONE', #9628, 5.000000000000000888 ) ;
#8041=CARTESIAN_POINT ( 'NONE',  ( 20.00000000000000000, 54.99999999999999289, -67.08203932499371547 ) ) ;
#8045=CARTESIAN_POINT ( 'NONE',  ( 69.53320273752072467, 19.33188093005041353, 28.10933780299437856 ) ) ;
#8047=AXIS2_PLACEMENT_3D ( 'NONE', #9101, #5384, #11056 ) ;
#8049=CARTESIAN_POINT ( 'NONE',  ( 72.61843774138908714, 45.00000000000009237, -18.75000000000000355 ) ) ;
#8053=CARTESIAN_POINT ( 'NONE',  ( 71.74731260882261097, 44.73211708709012413, 21.96902955818388392 ) ) ;
#8060=ADVANCED_FACE ( 'NONE', ( #7193 ), #10996, .T. ) ;
#8061=EDGE_CURVE ( 'NONE', #934, #6417, #2442, .T. ) ;
#8068=DIRECTION ( 'NONE',  ( -1.000000000000000000, -0.000000000000000000, -0.000000000000000000 ) ) ;
#8073=CARTESIAN_POINT ( 'NONE',  ( 13.70065104476912587, 28.13883518474186829, 73.73801000603624800 ) ) ;
#8075=EDGE_CURVE ( 'NONE', #712, #592, #9662, .T. ) ;
#8078=FACE_OUTER_BOUND ( 'NONE', #12001, .T. ) ;
#8091=CARTESIAN_POINT ( 'NONE',  ( 72.28523001630050260, 49.93187928610722537, -20.00612389586593309 ) ) ;
#8094=CARTESIAN_POINT ( 'NONE',  ( 170.0000000000011369, 30.00000000000008882, 25.00000000000000000 ) ) ;
#8096=VERTEX_POINT ( 'NONE', #50 ) ;
#8105=CARTESIAN_POINT ( 'NONE',  ( 74.29751312657262474, 18.66988058564614761, 24.83155917518388733 ) ) ;
#8107=ORIENTED_EDGE ( 'NONE', *, *, #1750, .T. ) ;
#8109=CARTESIAN_POINT ( 'NONE',  ( 76.23711339313383917, 15.46430896355019158, 22.12715364262389883 ) ) ;
#8113=CARTESIAN_POINT ( 'NONE',  ( 74.16198487146469631, 40.33897449742281083, 25.00000000000000000 ) ) ;
#8120=VECTOR ( 'NONE', #789, 1000.000000000000114 ) ;
#8122=ORIENTED_EDGE ( 'NONE', *, *, #2585, .F. ) ;
#8128=EDGE_CURVE ( 'NONE', #934, #3388, #6731, .T. ) ;
#8129=LINE ( 'NONE', #6213, #58 ) ;
#8140=ADVANCED_FACE ( 'NONE', ( #2057 ), #7881, .T. ) ;
#8144=DIRECTION ( 'NONE',  ( 1.000000000000000000, 0.000000000000000000, 0.000000000000000000 ) ) ;
#8145=CARTESIAN_POINT ( 'NONE',  ( 74.16198487095665826, 20.00000000000009237, -25.00000000000000000 ) ) ;
#8149=CARTESIAN_POINT ( 'NONE',  ( 145.0000000000011369, 67.07106781186550393, 20.00000000000000000 ) ) ;
#8150=ORIENTED_EDGE ( 'NONE', *, *, #7549, .F. ) ;
#8153=VERTEX_POINT ( 'NONE', #8587 ) ;
#8157=CARTESIAN_POINT ( 'NONE',  ( -1.190781129305471087, 30.00000000000008882, 65.00000000000000000 ) ) ;
#8158=CARTESIAN_POINT ( 'NONE',  ( -20.00000000000004263, 50.00000000000000000, 67.08203932499370126 ) ) ;
#8160=CARTESIAN_POINT ( 'NONE',  ( 20.00000000000000000, 7.965803112215716020, 67.08203932499371547 ) ) ;
#8163=CARTESIAN_POINT ( 'NONE',  ( 20.00000000000000000, 54.99999999999999289, -67.08203932499371547 ) ) ;
#8170=CARTESIAN_POINT ( 'NONE',  ( 71.59624044336385396, 15.53386596841878919, 22.48149205125783823 ) ) ;
#8176=ORIENTED_EDGE ( 'NONE', *, *, #9732, .F. ) ;
#8178=CARTESIAN_POINT ( 'NONE',  ( 71.43628325305886051, 49.01507604668937290, 22.85167202658856667 ) ) ;
#8179=ORIENTED_EDGE ( 'NONE', *, *, #8210, .T. ) ;
#8194=CARTESIAN_POINT ( 'NONE',  ( 13.11583011321536141, 25.39745421660067848, 73.84506090661903954 ) ) ;
#8197=CARTESIAN_POINT ( 'NONE',  ( 1.224646799147353059E-15, 110.0000000000000000, -9.999999999999998224 ) ) ;
#8200=CARTESIAN_POINT ( 'NONE',  ( 0.000000000000000000, 110.0000000000000000, -15.00000000000000000 ) ) ;
#8204=CARTESIAN_POINT ( 'NONE',  ( 165.0000000000011369, 225.0000000000000853, 20.00000000000000000 ) ) ;
#8206=ORIENTED_EDGE ( 'NONE', *, *, #9808, .T. ) ;
#8207=VECTOR ( 'NONE', #877, 1000.000000000000000 ) ;
#8210=EDGE_CURVE ( 'NONE', #3340, #5994, #6857, .T. ) ;
#8211=ORIENTED_EDGE ( 'NONE', *, *, #6836, .T. ) ;
#8221=DIRECTION ( 'NONE',  ( 3.469446951953613203E-16, 0.000000000000000000, 1.000000000000000000 ) ) ;
#8229=ORIENTED_EDGE ( 'NONE', *, *, #2123, .F. ) ;
#8241=ORIENTED_EDGE ( 'NONE', *, *, #6773, .F. ) ;
#8244=ADVANCED_FACE ( 'NONE', ( #1489 ), #11070, .T. ) ;
#8252=EDGE_CURVE ( 'NONE', #3388, #11037, #3730, .T. ) ;
#8263=VECTOR ( 'NONE', #5964, 1000.000000000000000 ) ;
#8266=AXIS2_PLACEMENT_3D ( 'NONE', #6670, #1934, #2234 ) ;
#8270=CARTESIAN_POINT ( 'NONE',  ( 69.65901248891714204, 17.35373687154389444, -27.79625982057084244 ) ) ;
#8272=EDGE_CURVE ( 'NONE', #6450, #8096, #550, .T. ) ;
#8273=VECTOR ( 'NONE', #3376, 1000.000000000000000 ) ;
#8277=EDGE_LOOP ( 'NONE', ( #11129, #4800, #8760, #2148 ) ) ;
#8281=LINE ( 'NONE', #11161, #4542 ) ;
#8283=VERTEX_POINT ( 'NONE', #7159 ) ;
#8291=ORIENTED_EDGE ( 'NONE', *, *, #10455, .F. ) ;
#8294=FACE_OUTER_BOUND ( 'NONE', #8896, .T. ) ;
#8298=FACE_OUTER_BOUND ( 'NONE', #5274, .T. ) ;
#8300=CARTESIAN_POINT ( 'NONE',  ( -16.19078112930547064, 29.48268919737577320, 73.23154106273422315 ) ) ;
#8303=CARTESIAN_POINT ( 'NONE',  ( -26.76795759904968364, 61.76795759904965877, 64.77864552555394084 ) ) ;
#8317=CARTESIAN_POINT ( 'NONE',  ( -12.80572322781401695, 39.54834576183792194, 73.90120587261097285 ) ) ;
#8322=CARTESIAN_POINT ( 'NONE',  ( 9.184850993605150311E-15, 50.00000000000000000, 75.00000000000001421 ) ) ;
#8324=ADVANCED_FACE ( 'NONE', ( #10835 ), #1365, .T. ) ;
#8329=DIRECTION ( 'NONE',  ( -1.000000000000000000, 0.000000000000000000, 0.000000000000000000 ) ) ;
#8337=CARTESIAN_POINT ( 'NONE',  ( 0.000000000000000000, 115.0000000000000000, 0.000000000000000000 ) ) ;
#8339=CARTESIAN_POINT ( 'NONE',  ( 2.020667218593133416E-14, 63.00000000000000000, 70.00000000000000000 ) ) ;
#8343=CARTESIAN_POINT ( 'NONE',  ( 0.000000000000000000, 63.00000000000000000, 0.000000000000000000 ) ) ;
#8356=LINE ( 'NONE', #6506, #7940 ) ;
#8357=CARTESIAN_POINT ( 'NONE',  ( -16.19078112930547064, 30.00000000000008882, 73.23154106273422315 ) ) ;
#8371=AXIS2_PLACEMENT_3D ( 'NONE', #5718, #4770, #1037 ) ;
#8372=VECTOR ( 'NONE', #1818, 1000.000000000000000 ) ;
#8374=CARTESIAN_POINT ( 'NONE',  ( 170.0000000000011369, 35.00000000000004974, -19.99999999999999645 ) ) ;
#8376=CARTESIAN_POINT ( 'NONE',  ( 0.000000000000000000, 20.00000000000009237, 25.00000000000000000 ) ) ;
#8387=CARTESIAN_POINT ( 'NONE',  ( 20.00000000000000355, 63.00000000000000000, 57.08203932499370836 ) ) ;
#8390=ADVANCED_FACE ( 'NONE', ( #6655 ), #3702, .T. ) ;
#8393=LINE ( 'NONE', #12335, #6093 ) ;
#8398=VERTEX_POINT ( 'NONE', #11215 ) ;
#8403=LINE ( 'NONE', #6359, #7337 ) ;
#8406=ORIENTED_EDGE ( 'NONE', *, *, #8682, .T. ) ;
#8410=CARTESIAN_POINT ( 'NONE',  ( -20.00000000000000355, 7.965803112215716020, -57.08203932499370836 ) ) ;
#8412=CARTESIAN_POINT ( 'NONE',  ( 145.0000000000011369, 230.0000000000000853, -20.00000000000000000 ) ) ;
#8418=CARTESIAN_POINT ( 'NONE',  ( 0.000000000000000000, 110.0000000000000000, 9.999999999999998224 ) ) ;
#8419=DIRECTION ( 'NONE',  ( 0.000000000000000000, 0.000000000000000000, 1.000000000000000000 ) ) ;
#8422=FACE_BOUND ( 'NONE', #6871, .T. ) ;
#8425=DIRECTION ( 'NONE',  ( 0.000000000000000000, -1.000000000000000000, 0.000000000000000000 ) ) ;
#8427=EDGE_CURVE ( 'NONE', #6026, #5348, #8393, .T. ) ;
#8429=ADVANCED_FACE ( 'NONE', ( #12153 ), #5481, .F. ) ;
#8433=AXIS2_PLACEMENT_3D ( 'NONE', #7037, #7226, #9832 ) ;
#8434=DIRECTION ( 'NONE',  ( 0.000000000000000000, 0.000000000000000000, 1.000000000000000000 ) ) ;
#8438=CARTESIAN_POINT ( 'NONE',  ( -5.124469781714441119, 44.48424997675835613, 74.82642711344708175 ) ) ;
#8440=ADVANCED_FACE ( 'NONE', ( #1737 ), #3218, .F. ) ;
#8446=AXIS2_PLACEMENT_3D ( 'NONE', #314, #4941, #10725 ) ;
#8452=DIRECTION ( 'NONE',  ( -1.000000000000000000, 0.000000000000000000, -0.000000000000000000 ) ) ;
#8459=DIRECTION ( 'NONE',  ( 0.000000000000000000, 0.000000000000000000, 1.000000000000000000 ) ) ;
#8461=EDGE_LOOP ( 'NONE', ( #5019, #2686, #2801, #690 ) ) ;
#8463=DIRECTION ( 'NONE',  ( 0.000000000000000000, 1.000000000000000000, 0.000000000000000000 ) ) ;
#8466=CARTESIAN_POINT ( 'NONE',  ( 140.0000000000011369, 67.07106781186550393, -20.00000000000000000 ) ) ;
#8472=EDGE_LOOP ( 'NONE', ( #2557, #2528, #9957, #12273 ) ) ;
#8475=EDGE_CURVE ( 'NONE', #3575, #7931, #602, .T. ) ;
#8476=VECTOR ( 'NONE', #6150, 1000.000000000000000 ) ;
#8487=VECTOR ( 'NONE', #652, 1000.000000000000000 ) ;
#8488=DIRECTION ( 'NONE',  ( 0.7071067811865464625, 0.7071067811865486830, -2.453269466693394184E-16 ) ) ;
#8507=CARTESIAN_POINT ( 'NONE',  ( 69.57792926911190534, 41.67137613650560013, -27.99850680361992517 ) ) ;
#8513=CARTESIAN_POINT ( 'NONE',  ( 74.38206444891756064, 18.35649441856873665, -24.72514820121006807 ) ) ;
#8514=ORIENTED_EDGE ( 'NONE', *, *, #4544, .T. ) ;
#8526=DIRECTION ( 'NONE',  ( -0.000000000000000000, 1.000000000000000000, -0.000000000000000000 ) ) ;
#8527=VERTEX_POINT ( 'NONE', #347 ) ;
#8531=EDGE_LOOP ( 'NONE', ( #6931, #2500, #1749 ) ) ;
#8536=AXIS2_PLACEMENT_3D ( 'NONE', #7801, #4814, #3878 ) ;
#8539=DIRECTION ( 'NONE',  ( 0.000000000000000000, -0.000000000000000000, -1.000000000000000000 ) ) ;
#8542=CARTESIAN_POINT ( 'NONE',  ( 77.45966692414835109, 50.00000000000008527, 20.00000000000000000 ) ) ;
#8545=EDGE_CURVE ( 'NONE', #4020, #2560, #7946, .T. ) ;
#8551=B_SPLINE_CURVE_WITH_KNOTS ( 'NONE', 3,
 ( #7091, #3351, #2345, #6152, #9820, #6033, #11650, #9942, #1418, #1234, #5041, #288, #10067, #3536, #11138, #9188, #3415, #604, #2537, #11955, #7212, #3473, #2597, #1543, #6403, #5346 ),
 .UNSPECIFIED., .F., .F.,
 ( 4, 2, 2, 2, 2, 2, 2, 2, 2, 2, 2, 2, 4 ),
 ( 1.055191096010040543E-17, 0.001946127227419493797, 0.002919190841129235166, 0.003892254454838976752, 0.005838381682258450382, 0.006811445295968177223, 0.007784508909677903196, 0.008757572523387630037, 0.009730636137097358612, 0.01167676336451680709, 0.01264982697822653740, 0.01362289059193626597, 0.01556901781935573700 ),
 .UNSPECIFIED. ) ;
#8558=FACE_OUTER_BOUND ( 'NONE', #4764, .T. ) ;
#8562=CYLINDRICAL_SURFACE ( 'NONE', #4191, 70.00000000000001421 ) ;
#8564=AXIS2_PLACEMENT_3D ( 'NONE', #4085, #6081, #1221 ) ;
#8567=CARTESIAN_POINT ( 'NONE',  ( 74.29751312657262474, 41.33011941435380976, -24.83155917518393352 ) ) ;
#8569=AXIS2_PLACEMENT_3D ( 'NONE', #3250, #7058, #10855 ) ;
#8573=CARTESIAN_POINT ( 'NONE',  ( 72.28042146285945080, 14.83791805334885439, -20.04664579644849098 ) ) ;
#8576=CYLINDRICAL_SURFACE ( 'NONE', #10537, 70.00000000000001421 ) ;
#8585=VERTEX_POINT ( 'NONE', #11009 ) ;
#8587=CARTESIAN_POINT ( 'NONE',  ( 0.000000000000000000, 50.00000000000000000, -75.00000000000001421 ) ) ;
#8591=EDGE_CURVE ( 'NONE', #5183, #3340, #1624, .T. ) ;
#8592=FACE_OUTER_BOUND ( 'NONE', #2990, .T. ) ;
#8595=VERTEX_POINT ( 'NONE', #794 ) ;
#8597=CARTESIAN_POINT ( 'NONE',  ( 145.0000000000011369, 230.0000000000000853, 20.00000000000000000 ) ) ;
#8598=CIRCLE ( 'NONE', #5429, 9.999999999999994671 ) ;
#8599=EDGE_CURVE ( 'NONE', #6043, #10619, #1130, .T. ) ;
#8601=ORIENTED_EDGE ( 'NONE', *, *, #6658, .T. ) ;
#8603=CARTESIAN_POINT ( 'NONE',  ( -8.008617612132468366, 16.62907246060994737, 74.57265862153481351 ) ) ;
#8604=ORIENTED_EDGE ( 'NONE', *, *, #6032, .F. ) ;
#8606=CARTESIAN_POINT ( 'NONE',  ( 70.40708232491708429, 13.43343575954947156, 25.84664880093517070 ) ) ;
#8607=ORIENTED_EDGE ( 'NONE', *, *, #8210, .F. ) ;
#8610=DIRECTION ( 'NONE',  ( -1.000000000000000000, 0.000000000000000000, -0.000000000000000000 ) ) ;
#8621=FACE_OUTER_BOUND ( 'NONE', #1038, .T. ) ;
#8626=DIRECTION ( 'NONE',  ( 0.000000000000000000, 1.000000000000000000, 0.000000000000000000 ) ) ;
#8630=CARTESIAN_POINT ( 'NONE',  ( 74.70719529697929318, 42.54354230980619889, -24.30790125104183019 ) ) ;
#8634=CONICAL_SURFACE ( 'NONE', #4465, 75.00000000000001421, 0.7853981633974427279 ) ;
#8636=CARTESIAN_POINT ( 'NONE',  ( 71.99731494076550575, 14.95993129310641123, -21.09170898384848414 ) ) ;
#8646=DIRECTION ( 'NONE',  ( -0.7071067811865513475, -0.7071067811865437980, -0.000000000000000000 ) ) ;
#8650=CARTESIAN_POINT ( 'NONE',  ( 1.734723475976807094E-14, 63.00000000000000000, 57.08203932499370836 ) ) ;
#8655=LINE ( 'NONE', #4932, #10447 ) ;
#8668=CARTESIAN_POINT ( 'NONE',  ( 140.0000000000011369, 225.0000000000000853, 20.00000000000000000 ) ) ;
#8672=CARTESIAN_POINT ( 'NONE',  ( 0.000000000000000000, 50.00000000000000000, 0.000000000000000000 ) ) ;
#8677=SPHERICAL_SURFACE ( 'NONE', #2788, 5.000000000000000000 ) ;
#8678=CARTESIAN_POINT ( 'NONE',  ( 72.32495769890022075, 14.83846616281870467, 19.87825060515873687 ) ) ;
#8682=EDGE_CURVE ( 'NONE', #8789, #6619, #6901, .T. ) ;
#8690=CARTESIAN_POINT ( 'NONE',  ( 170.0000000000011369, 225.0000000000000853, 25.00000000000000000 ) ) ;
#8695=CARTESIAN_POINT ( 'NONE',  ( 71.74671581198448678, 44.73114732258832760, -21.97107035890099169 ) ) ;
#8696=SURFACE_STYLE_USAGE ( .BOTH. , #1915 ) ;
#8700=CARTESIAN_POINT ( 'NONE',  ( 75.14265900998621817, 16.66197922908980544, -23.72616954495079256 ) ) ;
#8702=CARTESIAN_POINT ( 'NONE',  ( 0.000000000000000000, 45.00000000000008527, 0.000000000000000000 ) ) ;
#8707=EDGE_CURVE ( 'NONE', #6555, #7679, #4836, .T. ) ;
#8711=DIRECTION ( 'NONE',  ( 0.000000000000000000, 0.000000000000000000, -1.000000000000000000 ) ) ;
#8715=VERTEX_POINT ( 'NONE', #12321 ) ;
#8726=DIRECTION ( 'NONE',  ( 0.000000000000000000, 0.000000000000000000, 1.000000000000000000 ) ) ;
#8736=EDGE_CURVE ( 'NONE', #11474, #3822, #10689, .T. ) ;
#8741=B_SPLINE_CURVE_WITH_KNOTS ( 'NONE', 3,
 ( #5252, #7978, #5942, #6003, #4128, #11806, #3194, #5076, #9790, #9913, #2317, #2194, #9977, #10675, #1383, #7919, #5192, #8972 ),
 .UNSPECIFIED., .F., .F.,
 ( 4, 2, 2, 2, 2, 2, 2, 2, 4 ),
 ( 0.000000000000000000, 0.001070780962355597030, 0.002141561924711194061, 0.003212342887066791091, 0.004283123849422388121, 0.005353904811777984718, 0.006424685774133582182, 0.007495466736489179646, 0.008566247698844776243 ),
 .UNSPECIFIED. ) ;
#8747=CARTESIAN_POINT ( 'NONE',  ( 0.000000000000000000, 115.0000000000000000, 0.000000000000000000 ) ) ;
#8758=CIRCLE ( 'NONE', #7965, 25.00000000000000000 ) ;
#8759=CARTESIAN_POINT ( 'NONE',  ( 72.29800075079589305, 10.06258521785520976, -19.95946618966756958 ) ) ;
#8760=ORIENTED_EDGE ( 'NONE', *, *, #6468, .F. ) ;
#8770=ORIENTED_EDGE ( 'NONE', *, *, #5852, .F. ) ;
#8774=ORIENTED_EDGE ( 'NONE', *, *, #3560, .F. ) ;
#8777=AXIS2_PLACEMENT_3D ( 'NONE', #9908, #564, #5248 ) ;
#8779=CIRCLE ( 'NONE', #3421, 5.000000000000000888 ) ;
#8780=CARTESIAN_POINT ( 'NONE',  ( 13.80921887069452758, 30.00000000000009237, 65.00000000000000000 ) ) ;
#8786=ORIENTED_EDGE ( 'NONE', *, *, #10703, .T. ) ;
#8788=CYLINDRICAL_SURFACE ( 'NONE', #3280, 75.00000000000001421 ) ;
#8789=VERTEX_POINT ( 'NONE', #2839 ) ;
#8790=CARTESIAN_POINT ( 'NONE',  ( 165.0000000000011369, 225.0000000000000853, -20.00000000000000000 ) ) ;
#8799=EDGE_LOOP ( 'NONE', ( #8291, #9537, #2137, #10084 ) ) ;
#8800=ORIENTED_EDGE ( 'NONE', *, *, #1498, .F. ) ;
#8803=CIRCLE ( 'NONE', #4042, 75.00000000000001421 ) ;
#8805=EDGE_CURVE ( 'NONE', #8595, #7410, #4706, .T. ) ;
#8811=ORIENTED_EDGE ( 'NONE', *, *, #8252, .T. ) ;
#8818=CARTESIAN_POINT ( 'NONE',  ( 74.91301266955075278, 17.04453457915816728, -24.03638115575044409 ) ) ;
#8832=ORIENTED_EDGE ( 'NONE', *, *, #10642, .F. ) ;
#8836=FACE_OUTER_BOUND ( 'NONE', #1363, .T. ) ;
#8837=CARTESIAN_POINT ( 'NONE',  ( 72.61843774138907293, 50.00000000000000000, -18.75000000000000000 ) ) ;
#8843=CARTESIAN_POINT ( 'NONE',  ( 0.000000000000000000, 115.0000000000000000, 0.000000000000000000 ) ) ;
#8851=DIRECTION ( 'NONE',  ( 0.7071067811865513475, 0.7071067811865437980, 0.000000000000000000 ) ) ;
#8854=DIRECTION ( 'NONE',  ( 0.7071067811865486830, -0.7071067811865464625, 0.000000000000000000 ) ) ;
#8856=CARTESIAN_POINT ( 'NONE',  ( 71.26020304811973460, 11.28911591861274744, 23.39373652035272144 ) ) ;
#8857=AXIS2_PLACEMENT_3D ( 'NONE', #10760, #9939, #10943 ) ;
#8858=EDGE_CURVE ( 'NONE', #9381, #3427, #10273, .T. ) ;
#8860=AXIS2_PLACEMENT_3D ( 'NONE', #6220, #8488, #6570 ) ;
#8874=ADVANCED_FACE ( 'NONE', ( #4264 ), #9872, .F. ) ;
#8882=CARTESIAN_POINT ( 'NONE',  ( 20.00000000000000355, 7.965803112215716020, -57.08203932499370836 ) ) ;
#8890=EDGE_CURVE ( 'NONE', #5487, #10768, #9078, .T. ) ;
#8891=ORIENTED_EDGE ( 'NONE', *, *, #10112, .F. ) ;
#8895=DIRECTION ( 'NONE',  ( 0.000000000000000000, 0.000000000000000000, 1.000000000000000000 ) ) ;
#8896=EDGE_LOOP ( 'NONE', ( #7842, #10292, #4607, #4746 ) ) ;
#8898=DIRECTION ( 'NONE',  ( 0.000000000000000000, 0.000000000000000000, -1.000000000000000000 ) ) ;
#8901=ORIENTED_EDGE ( 'NONE', *, *, #9547, .T. ) ;
#8902=LINE ( 'NONE', #9082, #4579 ) ;
#8904=DIRECTION ( 'NONE',  ( -0.000000000000000000, -0.000000000000000000, 1.000000000000000000 ) ) ;
#8906=ORIENTED_EDGE ( 'NONE', *, *, #1891, .T. ) ;
#8907=CARTESIAN_POINT ( 'NONE',  ( 0.000000000000000000, -5.000000000000000000, 0.000000000000000000 ) ) ;
#8908=LINE ( 'NONE', #374, #8273 ) ;
#8909=VECTOR ( 'NONE', #9210, 1000.000000000000000 ) ;
#8911=CARTESIAN_POINT ( 'NONE',  ( -20.00000000000000355, 50.00000000000000000, -57.08203932499370836 ) ) ;
#8915=FACE_OUTER_BOUND ( 'NONE', #1555, .T. ) ;
#8916=CARTESIAN_POINT ( 'NONE',  ( 70.03799559100536953, 14.91291538047573439, 26.82731484558927093 ) ) ;
#8919=CARTESIAN_POINT ( 'NONE',  ( 76.05876219242703939, 15.60447527335573703, 22.40335076292606331 ) ) ;
#8920=CARTESIAN_POINT ( 'NONE',  ( 69.87020289360394543, 44.20576086388582127, -27.26117375607963922 ) ) ;
#8925=CARTESIAN_POINT ( 'NONE',  ( 71.59683363033870762, 44.46727110088187374, 22.47949853503603990 ) ) ;
#8926=EDGE_LOOP ( 'NONE', ( #1531, #1188, #7655 ) ) ;
#8929=DIRECTION ( 'NONE',  ( -0.000000000000000000, -1.000000000000000000, -0.000000000000000000 ) ) ;
#8930=EDGE_CURVE ( 'NONE', #4639, #592, #1925, .T. ) ;
#8933=VERTEX_POINT ( 'NONE', #3522 ) ;
#8934=AXIS2_PLACEMENT_3D ( 'NONE', #3301, #7163, #10023 ) ;
#8938=DIRECTION ( 'NONE',  ( 0.9682458365518543664, 0.000000000000000000, -0.2499999999999996947 ) ) ;
#8941=CARTESIAN_POINT ( 'NONE',  ( 140.0000000000011369, 67.07106781186550393, 25.00000000000000000 ) ) ;
#8942=LINE ( 'NONE', #9882, #9630 ) ;
#8947=VECTOR ( 'NONE', #6467, 1000.000000000000000 ) ;
#8952=DIRECTION ( 'NONE',  ( 0.000000000000000000, 0.000000000000000000, -1.000000000000000000 ) ) ;
#8957=ORIENTED_EDGE ( 'NONE', *, *, #10206, .T. ) ;
#8959=CIRCLE ( 'NONE', #3599, 5.000000000000000888 ) ;
#8961=VECTOR ( 'NONE', #2042, 1000.000000000000000 ) ;
#8966=EDGE_LOOP ( 'NONE', ( #9203, #7501, #4348, #11296 ) ) ;
#8967=DIRECTION ( 'NONE',  ( 0.000000000000000000, 1.000000000000000000, 0.000000000000000000 ) ) ;
#8968=CARTESIAN_POINT ( 'NONE',  ( 4.163799117101000559E-16, 109.0000000000000000, -3.399999999999999911 ) ) ;
#8972=CARTESIAN_POINT ( 'NONE',  ( 74.16198487095665826, 40.00000000000009237, -25.00000000000000000 ) ) ;
#8977=CARTESIAN_POINT ( 'NONE',  ( 74.21645788709501801, 19.16431193171542802, 24.93253696209799131 ) ) ;
#8985=ORIENTED_EDGE ( 'NONE', *, *, #11441, .F. ) ;
#8987=CARTESIAN_POINT ( 'NONE',  ( 74.16198487095664404, 40.00000000000009237, 25.00000000000000000 ) ) ;
#8990=LINE ( 'NONE', #10871, #9731 ) ;
#8997=CARTESIAN_POINT ( 'NONE',  ( 165.0000000000011369, 225.0000000000000853, 20.00000000000000000 ) ) ;
#9001=DIRECTION ( 'NONE',  ( 0.7071067811865495711, 0.7071067811865455743, -0.000000000000000000 ) ) ;
#9002=DIRECTION ( 'NONE',  ( 0.000000000000000000, 0.000000000000000000, -1.000000000000000000 ) ) ;
#9004=VECTOR ( 'NONE', #8463, 1000.000000000000000 ) ;
#9007=EDGE_CURVE ( 'NONE', #5882, #2768, #2760, .T. ) ;
#9019=CARTESIAN_POINT ( 'NONE',  ( 71.66825662749599246, 49.34246535461046790, -22.10769995529665977 ) ) ;
#9027=ORIENTED_EDGE ( 'NONE', *, *, #6008, .F. ) ;
#9029=CARTESIAN_POINT ( 'NONE',  ( -20.00000000000000355, 65.00000000000000000, 57.08203932499370836 ) ) ;
#9032=CARTESIAN_POINT ( 'NONE',  ( 0.000000000000000000, 50.00000000000000000, 0.000000000000000000 ) ) ;
#9033=DIRECTION ( 'NONE',  ( -3.469446951953613203E-16, 0.000000000000000000, -1.000000000000000000 ) ) ;
#9036=CARTESIAN_POINT ( 'NONE',  ( 70.29663099721912545, 13.81758329365315063, 26.14423569115638912 ) ) ;
#9039=AXIS2_PLACEMENT_3D ( 'NONE', #4109, #11907, #9955 ) ;
#9040=AXIS2_PLACEMENT_3D ( 'NONE', #9660, #11617, #8726 ) ;
#9046=CARTESIAN_POINT ( 'NONE',  ( 69.52686081700198883, 40.67794899483754278, 28.12499999881304191 ) ) ;
#9047=ORIENTED_EDGE ( 'NONE', *, *, #6697, .F. ) ;
#9055=ORIENTED_EDGE ( 'NONE', *, *, #4420, .T. ) ;
#9065=CARTESIAN_POINT ( 'NONE',  ( 0.000000000000000000, 115.0000000000000000, 0.000000000000000000 ) ) ;
#9072=VERTEX_POINT ( 'NONE', #10 ) ;
#9074=EDGE_CURVE ( 'NONE', #10619, #10742, #9681, .T. ) ;
#9078=CIRCLE ( 'NONE', #11094, 70.00000000000001421 ) ;
#9080=EDGE_CURVE ( 'NONE', #3926, #834, #2884, .T. ) ;
#9081=VERTEX_POINT ( 'NONE', #194 ) ;
#9082=CARTESIAN_POINT ( 'NONE',  ( 150.0000000000010800, 15.00000000000008882, -19.99999999999999645 ) ) ;
#9089=CARTESIAN_POINT ( 'NONE',  ( 72.28523001630050260, 10.06812071389296293, 20.00612389586592954 ) ) ;
#9096=CARTESIAN_POINT ( 'NONE',  ( 74.16874958671132845, 19.66594046503222515, 24.99164682819348471 ) ) ;
#9097=ORIENTED_EDGE ( 'NONE', *, *, #11041, .F. ) ;
#9098=CIRCLE ( 'NONE', #10904, 14.99999999999999822 ) ;
#9100=CARTESIAN_POINT ( 'NONE',  ( 77.45966692414835109, 45.00000000000009237, -20.00000000000000355 ) ) ;
#9101=CARTESIAN_POINT ( 'NONE',  ( 74.16198487095665826, 20.00000000000009237, 30.00000000000000355 ) ) ;
#9104=CARTESIAN_POINT ( 'NONE',  ( 70.80917463421374691, 40.85568721397550007, 24.94686153084717617 ) ) ;
#9123=CARTESIAN_POINT ( 'NONE',  ( 13.80921887069452758, 30.00000000000009237, 73.71774192269630532 ) ) ;
#9125=DIRECTION ( 'NONE',  ( 1.224646799147352961E-16, 0.000000000000000000, -1.000000000000000000 ) ) ;
#9128=EDGE_CURVE ( 'NONE', #5113, #9199, #7809, .T. ) ;
#9130=ORIENTED_EDGE ( 'NONE', *, *, #3582, .F. ) ;
#9134=DIRECTION ( 'NONE',  ( -0.000000000000000000, 1.000000000000000000, -0.000000000000000000 ) ) ;
#9148=DIRECTION ( 'NONE',  ( -0.000000000000000000, 1.000000000000000000, -0.000000000000000000 ) ) ;
#9156=DIRECTION ( 'NONE',  ( 1.564230817409691233E-15, 0.000000000000000000, -1.000000000000000000 ) ) ;
#9167=CARTESIAN_POINT ( 'NONE',  ( 0.000000000000000000, 225.0000000000000853, -25.00000000000000000 ) ) ;
#9173=TOROIDAL_SURFACE ( 'NONE', #7968, 65.00000000000001421, 5.000000000000000000 ) ;
#9178=VERTEX_POINT ( 'NONE', #134 ) ;
#9180=DIRECTION ( 'NONE',  ( 0.000000000000000000, 0.000000000000000000, -1.000000000000000000 ) ) ;
#9183=DIRECTION ( 'NONE',  ( -0.7071067811865511255, -0.7071067811865440200, 9.813077866773545180E-16 ) ) ;
#9188=CARTESIAN_POINT ( 'NONE',  ( 70.26686370603788134, 13.95206716814361236, -26.22231631056802925 ) ) ;
#9193=( BOUNDED_SURFACE ( )  B_SPLINE_SURFACE ( 3, 2, ( 
 ( #4201, #7009, #8987 ),
 ( #9046, #2385, #8113 ),
 ( #4139, #9104, #3455 ),
 ( #7258, #11819, #7129 ),
 ( #393, #6321, #10927 ),
 ( #3262, #6197, #1460 ),
 ( #10106, #7069, #520 ),
 ( #3329, #10866, #11938 ),
 ( #6261, #10804, #1582 ),
 ( #4260, #2328, #9865 ),
 ( #6135, #11879, #5267 ),
 ( #9925, #9989, #1397 ),
 ( #3207, #580, #4379 ),
 ( #5387, #2267, #5206 ),
 ( #4318, #8925, #3393 ),
 ( #455, #7191, #10994 ),
 ( #6074, #8053, #11059 ),
 ( #2455, #10049, #1524 ),
 ( #8178, #2521, #12000 ),
 ( #333, #7930, #11754 ),
 ( #1339, #5147, #1646 ),
 ( #10171, #7443, #7322 ),
 ( #2637, #10420, #6510 ),
 ( #1709, #5518, #9294 ),
 ( #12306, #715, #6625 ),
 ( #1766, #11310, #9231 ) ),
 .UNSPECIFIED., .F., .F., .F. ) 
 B_SPLINE_SURFACE_WITH_KNOTS ( ( 4, 2, 2, 2, 2, 2, 2, 2, 2, 2, 2, 2, 4 ),
 ( 3, 3 ),
 ( 0.006382978049045527277, 0.008387885753076827766, 0.009390339605092477143, 0.01039279345710812652, 0.01239770116113942701, 0.01340015501315507812, 0.01440260886517072750, 0.01540506271718637861, 0.01640751656920202972, 0.01841242427323332848, 0.01941487812524897785, 0.02041733197726462723, 0.02242223968129592598 ),
 ( 0.000000000000000000, 1.000000000000000000 ),
 .UNSPECIFIED. ) 
 GEOMETRIC_REPRESENTATION_ITEM ( )  RATIONAL_B_SPLINE_SURFACE ( (
 ( 1.000000000000000000, 0.8291561975888499525, 1.000000000000000000),
 ( 1.000000000000000000, 0.8291533992853559187, 1.000000000000000000),
 ( 1.000000000000000000, 0.8281244206746621872, 1.000000000000000000),
 ( 1.000000000000000000, 0.8251351734919457614, 1.000000000000000000),
 ( 1.000000000000000000, 0.8238971056969668361, 1.000000000000000000),
 ( 1.000000000000000000, 0.8209398665854361621, 1.000000000000000000),
 ( 1.000000000000000000, 0.8192278287709440221, 1.000000000000000000),
 ( 1.000000000000000000, 0.8135208904818045372, 1.000000000000000000),
 ( 1.000000000000000000, 0.8089311958808242942, 1.000000000000000000),
 ( 1.000000000000000000, 0.8010155071010776062, 1.000000000000000000),
 ( 1.000000000000000000, 0.7981992791122975994, 1.000000000000000000),
 ( 1.000000000000000000, 0.7923673440970770976, 1.000000000000000000),
 ( 1.000000000000000000, 0.7893380284541040570, 1.000000000000000000),
 ( 1.000000000000000000, 0.7830853791992800073, 1.000000000000000000),
 ( 1.000000000000000000, 0.7798619748040830357, 1.000000000000000000),
 ( 1.000000000000000000, 0.7732488416061537029, 1.000000000000000000),
 ( 1.000000000000000000, 0.7698413672833309684, 1.000000000000000000),
 ( 1.000000000000000000, 0.7595660318242437592, 1.000000000000000000),
 ( 1.000000000000000000, 0.7526475626048493295, 1.000000000000000000),
 ( 1.000000000000000000, 0.7423381171274799906, 1.000000000000000000),
 ( 1.000000000000000000, 0.7389127554685368526, 1.000000000000000000),
 ( 1.000000000000000000, 0.7321112719851028405, 1.000000000000000000),
 ( 1.000000000000000000, 0.7287565628962664466, 1.000000000000000000),
 ( 1.000000000000000000, 0.7189979416187094463, 1.000000000000000000),
 ( 1.000000000000000000, 0.7128432726192635016, 1.000000000000000000),
 ( 1.000000000000000000, 0.7071067811865476838, 1.000000000000000000) ) ) 
 REPRESENTATION_ITEM ( '' )  SURFACE ( )  );
#9199=VERTEX_POINT ( 'NONE', #1951 ) ;
#9200=AXIS2_PLACEMENT_3D ( 'NONE', #4860, #172, #2171 ) ;
#9202=PLANE ( 'NONE',  #4980 ) ;
#9203=ORIENTED_EDGE ( 'NONE', *, *, #9457, .T. ) ;
#9205=EDGE_CURVE ( 'NONE', #6384, #9696, #5763, .T. ) ;
#9210=DIRECTION ( 'NONE',  ( -0.000000000000000000, -1.000000000000000000, -0.000000000000000000 ) ) ;
#9211=CARTESIAN_POINT ( 'NONE',  ( -1.190781129305471087, 30.00000000000008882, 75.00000000000001421 ) ) ;
#9215=ORIENTED_EDGE ( 'NONE', *, *, #9281, .T. ) ;
#9219=AXIS2_PLACEMENT_3D ( 'NONE', #4273, #728, #11130 ) ;
#9226=LINE ( 'NONE', #711, #7264 ) ;
#9228=VERTEX_POINT ( 'NONE', #7057 ) ;
#9229=AXIS2_PLACEMENT_3D ( 'NONE', #3789, #5850, #11401 ) ;
#9231=CARTESIAN_POINT ( 'NONE',  ( 77.45966692414835109, 45.00000000000009237, 20.00000000000000711 ) ) ;
#9233=CARTESIAN_POINT ( 'NONE',  ( 149.1421356237320026, 17.07106781186555722, -24.99999999999998934 ) ) ;
#9250=CARTESIAN_POINT ( 'NONE',  ( -16.19078112930547064, 30.00000000000008882, 73.23154106273422315 ) ) ;
#9251=ADVANCED_FACE ( 'NONE', ( #321 ), #7118, .T. ) ;
#9252=CARTESIAN_POINT ( 'NONE',  ( 13.63461413510340670, 27.67039418665449446, 73.75028910564438434 ) ) ;
#9258=DIRECTION ( 'NONE',  ( -0.000000000000000000, -1.000000000000000000, -0.000000000000000000 ) ) ;
#9259=VECTOR ( 'NONE', #8952, 1000.000000000000000 ) ;
#9263=CARTESIAN_POINT ( 'NONE',  ( 74.58021194344081550, 17.74117554919819284, -24.47298709600785571 ) ) ;
#9276=EDGE_LOOP ( 'NONE', ( #10937, #445, #312, #1707, #10659, #5166, #11887 ) ) ;
#9281=EDGE_CURVE ( 'NONE', #4428, #9777, #8741, .T. ) ;
#9291=CARTESIAN_POINT ( 'NONE',  ( 72.61843774138907293, 50.00000000000000000, 18.75000000000000000 ) ) ;
#9294=CARTESIAN_POINT ( 'NONE',  ( 77.11786746747833377, 44.96870739097081326, 20.64504863446540384 ) ) ;
#9304=EDGE_CURVE ( 'NONE', #10742, #8153, #4517, .T. ) ;
#9305=EDGE_CURVE ( 'NONE', #3388, #9777, #4245, .T. ) ;
#9312=CARTESIAN_POINT ( 'NONE',  ( -15.76722741620018731, 33.57691821622091766, 73.32398149152362521 ) ) ;
#9314=DIRECTION ( 'NONE',  ( 0.000000000000000000, 0.000000000000000000, -1.000000000000000000 ) ) ;
#9319=EDGE_LOOP ( 'NONE', ( #11540, #4754, #8211, #3424 ) ) ;
#9322=CARTESIAN_POINT ( 'NONE',  ( 70.79098555864042908, 20.00000000000008882, -24.99999999999999645 ) ) ;
#9327=ORIENTED_EDGE ( 'NONE', *, *, #8858, .T. ) ;
#9334=ORIENTED_EDGE ( 'NONE', *, *, #3285, .T. ) ;
#9339=LINE ( 'NONE', #1868, #3896 ) ;
#9340=DIRECTION ( 'NONE',  ( -0.9682458365518540333, -4.961309141293670183E-14, -0.2500000000000003331 ) ) ;
#9344=CARTESIAN_POINT ( 'NONE',  ( 69.52686081652184669, 20.00000000000009237, 28.12500000000000000 ) ) ;
#9350=CARTESIAN_POINT ( 'NONE',  ( 69.76162866618027181, 43.49853569900138694, 27.53780242413599666 ) ) ;
#9351=ORIENTED_EDGE ( 'NONE', *, *, #12134, .F. ) ;
#9358=DIRECTION ( 'NONE',  ( 0.000000000000000000, 0.000000000000000000, 1.000000000000000000 ) ) ;
#9362=ORIENTED_EDGE ( 'NONE', *, *, #937, .F. ) ;
#9374=CARTESIAN_POINT ( 'NONE',  ( -15.13490964629960978, 35.55200036032155708, 73.45732584901404039 ) ) ;
#9381=VERTEX_POINT ( 'NONE', #1634 ) ;
#9391=FACE_OUTER_BOUND ( 'NONE', #7434, .T. ) ;
#9395=CARTESIAN_POINT ( 'NONE',  ( 4.163799117101000559E-16, 115.0000000000000000, -3.399999999999999911 ) ) ;
#9400=CARTESIAN_POINT ( 'NONE',  ( 9.450654096908945471E-15, 44.95265997413478942, 75.00000000000001421 ) ) ;
#9411=CARTESIAN_POINT ( 'NONE',  ( 72.28493664348427217, 49.93201633561922392, 20.00732221823095713 ) ) ;
#9422=FACE_OUTER_BOUND ( 'NONE', #5459, .T. ) ;
#9425=AXIS2_PLACEMENT_3D ( 'NONE', #9065, #7889, #9002 ) ;
#9429=LINE ( 'NONE', #5774, #2236 ) ;
#9439=CARTESIAN_POINT ( 'NONE',  ( 69.72804008650257401, 43.29323253992120613, -27.62368211345594204 ) ) ;
#9441=DIRECTION ( 'NONE',  ( -1.000000000000000000, 0.000000000000000000, 0.000000000000000000 ) ) ;
#9442=VERTEX_POINT ( 'NONE', #3624 ) ;
#9446=CARTESIAN_POINT ( 'NONE',  ( 70.96239324365633649, 17.73867115851379950, -24.49110472308180064 ) ) ;
#9448=( GEOMETRIC_REPRESENTATION_CONTEXT ( 3 ) GLOBAL_UNCERTAINTY_ASSIGNED_CONTEXT ( ( #11888 ) ) GLOBAL_UNIT_ASSIGNED_CONTEXT ( ( #9501, #7646, #4844 ) ) REPRESENTATION_CONTEXT ( 'NONE', 'WORKASPACE' ) );
#9452=ORIENTED_EDGE ( 'NONE', *, *, #10991, .T. ) ;
#9456=ORIENTED_EDGE ( 'NONE', *, *, #7342, .F. ) ;
#9457=EDGE_CURVE ( 'NONE', #5052, #8595, #3027, .T. ) ;
#9461=VECTOR ( 'NONE', #9555, 1000.000000000000000 ) ;
#9464=ORIENTED_EDGE ( 'NONE', *, *, #3782, .T. ) ;
#9468=CARTESIAN_POINT ( 'NONE',  ( 0.000000000000000000, -10.00000000000000000, 0.000000000000000000 ) ) ;
#9470=ORIENTED_EDGE ( 'NONE', *, *, #8545, .F. ) ;
#9474=VERTEX_POINT ( 'NONE', #7178 ) ;
#9480=ORIENTED_EDGE ( 'NONE', *, *, #6024, .F. ) ;
#9483=CARTESIAN_POINT ( 'NONE',  ( 138.5355339059338462, 63.53553390593273775, -20.00000000000000000 ) ) ;
#9487=ORIENTED_EDGE ( 'NONE', *, *, #9457, .F. ) ;
#9489=CARTESIAN_POINT ( 'NONE',  ( 0.000000000000000000, -5.000000000000000000, 0.000000000000000000 ) ) ;
#9490=VERTEX_POINT ( 'NONE', #1572 ) ;
#9498=EDGE_CURVE ( 'NONE', #3728, #357, #3934, .T. ) ;
#9499=EDGE_CURVE ( 'NONE', #592, #4639, #6211, .T. ) ;
#9500=CARTESIAN_POINT ( 'NONE',  ( 74.16198487097054226, 40.16707677251596209, -25.00000000000000000 ) ) ;
#9501=( LENGTH_UNIT ( ) NAMED_UNIT ( * ) SI_UNIT ( .MILLI., .METRE. ) );
#9503=VECTOR ( 'NONE', #8646, 1000.000000000000000 ) ;
#9507=CARTESIAN_POINT ( 'NONE',  ( 70.03362437693311904, 14.90552201415263767, -26.84082993662185501 ) ) ;
#9508=ORIENTED_EDGE ( 'NONE', *, *, #3384, .T. ) ;
#9518=LINE ( 'NONE', #7841, #4641 ) ;
#9527=EDGE_LOOP ( 'NONE', ( #5803, #8150, #7652, #10057 ) ) ;
#9535=LINE ( 'NONE', #1375, #10131 ) ;
#9537=ORIENTED_EDGE ( 'NONE', *, *, #5190, .F. ) ;
#9539=CARTESIAN_POINT ( 'NONE',  ( -20.00000000000000000, 63.00000000000000000, -67.08203932499371547 ) ) ;
#9541=LINE ( 'NONE', #4821, #9623 ) ;
#9542=CARTESIAN_POINT ( 'NONE',  ( 20.00000000000000355, 7.965803112215716020, 57.08203932499370836 ) ) ;
#9547=EDGE_CURVE ( 'NONE', #9228, #9696, #6674, .T. ) ;
#9555=DIRECTION ( 'NONE',  ( -0.000000000000000000, 1.000000000000000000, -0.000000000000000000 ) ) ;
#9556=ORIENTED_EDGE ( 'NONE', *, *, #2050, .F. ) ;
#9557=DIRECTION ( 'NONE',  ( -1.000000000000000000, 0.000000000000000000, 0.000000000000000000 ) ) ;
#9562=CARTESIAN_POINT ( 'NONE',  ( 0.000000000000000000, 0.000000000000000000, 0.000000000000000000 ) ) ;
#9566=CARTESIAN_POINT ( 'NONE',  ( 75.13748311126856549, 43.33995240362821733, -23.73500236559034704 ) ) ;
#9567=CARTESIAN_POINT ( 'NONE',  ( 135.0000000000011084, 67.07106781186550393, -19.99999999999999645 ) ) ;
#9568=AXIS2_PLACEMENT_3D ( 'NONE', #2810, #6614, #3809 ) ;
#9572=CARTESIAN_POINT ( 'NONE',  ( 76.84714931290172046, 15.12440032299506143, -21.12007276954078350 ) ) ;
#9578=DIRECTION ( 'NONE',  ( 0.000000000000000000, 0.000000000000000000, 1.000000000000000000 ) ) ;
#9587=CARTESIAN_POINT ( 'NONE',  ( -16.19078112930547064, 30.00000000000008882, 75.00000000000001421 ) ) ;
#9600=CARTESIAN_POINT ( 'NONE',  ( 75.00000000000001421, 20.00000000000009237, -19.99999999999999645 ) ) ;
#9602=DIRECTION ( 'NONE',  ( 0.000000000000000000, 0.000000000000000000, -1.000000000000000000 ) ) ;
#9603=CARTESIAN_POINT ( 'NONE',  ( 69.90350624952220926, 15.60330682347095710, 27.17578603812306426 ) ) ;
#9610=CARTESIAN_POINT ( 'NONE',  ( 77.45966692414835109, 15.00000000000008882, 20.00000000000000355 ) ) ;
#9611=ORIENTED_EDGE ( 'NONE', *, *, #3757, .T. ) ;
#9616=ORIENTED_EDGE ( 'NONE', *, *, #3877, .T. ) ;
#9617=CARTESIAN_POINT ( 'NONE',  ( 142.0710678118665555, 59.99999999999998579, -20.00000000000000000 ) ) ;
#9619=DIRECTION ( 'NONE',  ( 1.564230817409691233E-15, 0.000000000000000000, -1.000000000000000000 ) ) ;
#9623=VECTOR ( 'NONE', #8610, 1000.000000000000000 ) ;
#9624=SURFACE_STYLE_USAGE ( .BOTH. , #12327 ) ;
#9626=CARTESIAN_POINT ( 'NONE',  ( 71.69575657208368114, 49.37823943430655049, -22.01828877003865514 ) ) ;
#9628=AXIS2_PLACEMENT_3D ( 'NONE', #8790, #10669, #9720 ) ;
#9630=VECTOR ( 'NONE', #10699, 1000.000000000000000 ) ;
#9636=ORIENTED_EDGE ( 'NONE', *, *, #6836, .F. ) ;
#9642=CARTESIAN_POINT ( 'NONE',  ( 76.59271415824169082, 44.76269180811209480, 21.55336028430496143 ) ) ;
#9647=EDGE_CURVE ( 'NONE', #9199, #1231, #6470, .T. ) ;
#9660=CARTESIAN_POINT ( 'NONE',  ( 145.0000000000011369, 225.0000000000000853, -20.00000000000000000 ) ) ;
#9661=EDGE_LOOP ( 'NONE', ( #7041, #644, #7752, #615 ) ) ;
#9662=CIRCLE ( 'NONE', #8266, 4.999999999999997335 ) ;
#9665=VERTEX_POINT ( 'NONE', #8200 ) ;
#9668=DIRECTION ( 'NONE',  ( 0.000000000000000000, 0.000000000000000000, -1.000000000000000000 ) ) ;
#9670=DIRECTION ( 'NONE',  ( 0.000000000000000000, 0.000000000000000000, -1.000000000000000000 ) ) ;
#9674=SHAPE_REPRESENTATION ( 'Die-Cast Base Motor Housing', ( #1612 ), #10763 ) ;
#9676=CARTESIAN_POINT ( 'NONE',  ( 75.00000000000001421, 15.00000000000008882, 25.00000000000000000 ) ) ;
#9681=CIRCLE ( 'NONE', #7700, 75.00000000000001421 ) ;
#9685=FILL_AREA_STYLE ('',( #155 ) ) ;
#9687=ORIENTED_EDGE ( 'NONE', *, *, #3487, .F. ) ;
#9689=ADVANCED_FACE ( 'NONE', ( #12270 ), #10073, .T. ) ;
#9693=ORIENTED_EDGE ( 'NONE', *, *, #5125, .F. ) ;
#9695=CARTESIAN_POINT ( 'NONE',  ( 72.32585155008061406, 14.83851532874689738, -19.87486525338129795 ) ) ;
#9696=VERTEX_POINT ( 'NONE', #8387 ) ;
#9697=DIRECTION ( 'NONE',  ( -4.440892098500626162E-15, 0.000000000000000000, 1.000000000000000000 ) ) ;
#9698=CARTESIAN_POINT ( 'NONE',  ( 165.0000000000011369, 225.0000000000000853, -25.00000000000000000 ) ) ;
#9702=ORIENTED_EDGE ( 'NONE', *, *, #5216, .F. ) ;
#9708=VERTEX_POINT ( 'NONE', #6285 ) ;
#9710=CARTESIAN_POINT ( 'NONE',  ( 20.00000000000000000, 50.00000000000000000, 67.08203932499371547 ) ) ;
#9711=ORIENTED_EDGE ( 'NONE', *, *, #10494, .F. ) ;
#9718=CARTESIAN_POINT ( 'NONE',  ( 0.000000000000000000, 40.00000000000009237, -25.00000000000000000 ) ) ;
#9720=DIRECTION ( 'NONE',  ( 0.000000000000000000, 0.000000000000000000, -1.000000000000000000 ) ) ;
#9721=CARTESIAN_POINT ( 'NONE',  ( 117.9289321881355193, 50.00000000000008527, -19.99999999999999645 ) ) ;
#9722=VERTEX_POINT ( 'NONE', #7283 ) ;
#9731=VECTOR ( 'NONE', #211, 1000.000000000000000 ) ;
#9732=EDGE_CURVE ( 'NONE', #2354, #9722, #5471, .T. ) ;
#9735=CARTESIAN_POINT ( 'NONE',  ( 170.0000000000011369, 35.00000000000006395, 22.92893218813452449 ) ) ;
#9736=CARTESIAN_POINT ( 'NONE',  ( 13.80921887069452758, 30.92976843375813445, 73.71774192269630532 ) ) ;
#9740=PLANE ( 'NONE',  #5197 ) ;
#9758=AXIS2_PLACEMENT_3D ( 'NONE', #3044, #4982, #9578 ) ;
#9759=LINE ( 'NONE', #1480, #280 ) ;
#9761=PRODUCT ( 'Die-Cast Base Motor Housing', 'Die-Cast Base Motor Housing', '', ( #2935 ) ) ;
#9770=EDGE_CURVE ( 'NONE', #3822, #5348, #8779, .T. ) ;
#9772=EDGE_LOOP ( 'NONE', ( #5333, #9470, #6541, #521 ) ) ;
#9777=VERTEX_POINT ( 'NONE', #4335 ) ;
#9780=CIRCLE ( 'NONE', #1211, 70.00000000000001421 ) ;
#9783=CARTESIAN_POINT ( 'NONE',  ( -3.619653695503104451, 15.18885885628891863, 74.91437445603884271 ) ) ;
#9787=EDGE_CURVE ( 'NONE', #9178, #3388, #3815, .T. ) ;
#9790=CARTESIAN_POINT ( 'NONE',  ( 75.53289395085349156, 43.87018216231679446, -23.18166983250910818 ) ) ;
#9791=LINE ( 'NONE', #322, #3795 ) ;
#9796=CARTESIAN_POINT ( 'NONE',  ( 71.74671581198677472, 15.26885267741330132, 21.97107035890156013 ) ) ;
#9800=ORIENTED_EDGE ( 'NONE', *, *, #2441, .F. ) ;
#9802=LINE ( 'NONE', #5772, #9461 ) ;
#9803=ORIENTED_EDGE ( 'NONE', *, *, #582, .T. ) ;
#9806=CARTESIAN_POINT ( 'NONE',  ( 0.000000000000000000, 65.00000000000000000, 0.000000000000000000 ) ) ;
#9808=EDGE_CURVE ( 'NONE', #6417, #8096, #5409, .T. ) ;
#9819=CIRCLE ( 'NONE', #6083, 15.00000000000000000 ) ;
#9820=CARTESIAN_POINT ( 'NONE',  ( 71.93323519045088688, 10.35045604464705349, -21.22984507177766034 ) ) ;
#9824=AXIS2_PLACEMENT_3D ( 'NONE', #714, #5266, #9924 ) ;
#9829=CARTESIAN_POINT ( 'NONE',  ( 4.163799117101000559E-16, 109.0000000000000000, -3.399999999999999911 ) ) ;
#9831=VERTEX_POINT ( 'NONE', #7148 ) ;
#9832=DIRECTION ( 'NONE',  ( 1.000000000000000000, 0.000000000000000000, 0.000000000000000000 ) ) ;
#9834=VECTOR ( 'NONE', #2056, 1000.000000000000000 ) ;
#9843=CARTESIAN_POINT ( 'NONE',  ( 0.000000000000000000, 10.00000000000017586, 0.000000000000000000 ) ) ;
#9845=ORIENTED_EDGE ( 'NONE', *, *, #800, .F. ) ;
#9848=DIRECTION ( 'NONE',  ( 0.7071067811865495711, 0.7071067811865455743, -0.000000000000000000 ) ) ;
#9855=CARTESIAN_POINT ( 'NONE',  ( 70.79098555865897424, 19.78735728330005372, 24.99999999997159961 ) ) ;
#9856=VECTOR ( 'NONE', #3223, 1000.000000000000000 ) ;
#9859=ORIENTED_EDGE ( 'NONE', *, *, #2623, .F. ) ;
#9861=CARTESIAN_POINT ( 'NONE',  ( 75.73945001075168193, 44.09015450245603063, -22.88037593554885518 ) ) ;
#9864=DIRECTION ( 'NONE',  ( -0.000000000000000000, -1.000000000000000000, -0.000000000000000000 ) ) ;
#9865=CARTESIAN_POINT ( 'NONE',  ( 74.91301266955075278, 42.95546542084321118, 24.03638115574963052 ) ) ;
#9868=VECTOR ( 'NONE', #5311, 999.9999999999998863 ) ;
#9869=DIRECTION ( 'NONE',  ( -0.000000000000000000, 1.000000000000000000, -0.000000000000000000 ) ) ;
#9872=CONICAL_SURFACE ( 'NONE', #942, 3.399999999999999911, 1.029744258676658974 ) ;
#9874=ORIENTED_EDGE ( 'NONE', *, *, #2583, .T. ) ;
#9876=ADVANCED_FACE ( 'NONE', ( #11328 ), #1728, .T. ) ;
#9877=AXIS2_PLACEMENT_3D ( 'NONE', #5136, #8851, #3379 ) ;
#9881=CARTESIAN_POINT ( 'NONE',  ( 9.450654096908945471E-15, 44.95265997413478942, 75.00000000000001421 ) ) ;
#9882=CARTESIAN_POINT ( 'NONE',  ( 140.0000000000011369, 225.0000000000000853, 25.00000000000000000 ) ) ;
#9894=CARTESIAN_POINT ( 'NONE',  ( 74.62285592809365653, 17.63426063501363927, -24.41804092124679570 ) ) ;
#9895=ORIENTED_EDGE ( 'NONE', *, *, #2955, .T. ) ;
#9906=LINE ( 'NONE', #561, #6236 ) ;
#9908=CARTESIAN_POINT ( 'NONE',  ( -1.190781129305471087, 30.00000000000008882, 75.00000000000001421 ) ) ;
#9913=CARTESIAN_POINT ( 'NONE',  ( 75.20175883194669098, 43.43544396156184462, -23.64678730934253537 ) ) ;
#9918=CARTESIAN_POINT ( 'NONE',  ( 70.81305327821827689, 19.15123444475166181, 24.93520811514207836 ) ) ;
#9920=ORIENTED_EDGE ( 'NONE', *, *, #2843, .T. ) ;
#9923=EDGE_LOOP ( 'NONE', ( #4043, #7954, #2240, #8770 ) ) ;
#9924=DIRECTION ( 'NONE',  ( 0.000000000000000000, 0.000000000000000000, -1.000000000000000000 ) ) ;
#9925=CARTESIAN_POINT ( 'NONE',  ( 70.44624282194196496, 46.67604154196500588, 25.73656789697686165 ) ) ;
#9933=EDGE_LOOP ( 'NONE', ( #2735, #5733 ) ) ;
#9939=DIRECTION ( 'NONE',  ( 1.000000000000000000, -0.000000000000000000, 0.000000000000000000 ) ) ;
#9941=CARTESIAN_POINT ( 'NONE',  ( 165.0000000000011369, 225.0000000000000853, 20.00000000000000000 ) ) ;
#9942=CARTESIAN_POINT ( 'NONE',  ( 71.39985347493269785, 11.04390332592970481, -22.96547907468803373 ) ) ;
#9947=ORIENTED_EDGE ( 'NONE', *, *, #10347, .F. ) ;
#9953=EDGE_LOOP ( 'NONE', ( #2793, #10449, #5186 ) ) ;
#9955=DIRECTION ( 'NONE',  ( -1.000000000000000000, 0.000000000000000000, 0.000000000000000000 ) ) ;
#9957=ORIENTED_EDGE ( 'NONE', *, *, #3582, .T. ) ;
#9958=CYLINDRICAL_SURFACE ( 'NONE', #79, 5.000000000000000888 ) ;
#9959=CARTESIAN_POINT ( 'NONE',  ( 0.000000000000000000, 40.00000000000009237, -20.00000000000000000 ) ) ;
#9960=EDGE_CURVE ( 'NONE', #9490, #3926, #9780, .T. ) ;
#9963=AXIS2_PLACEMENT_3D ( 'NONE', #7624, #10300, #1888 ) ;
#9964=EDGE_CURVE ( 'NONE', #5388, #1747, #202, .T. ) ;
#9967=DIRECTION ( 'NONE',  ( 2.213536252433181072E-16, 0.000000000000000000, 1.000000000000000000 ) ) ;
#9968=DIRECTION ( 'NONE',  ( 1.000000000000000000, 0.000000000000000000, -0.000000000000000000 ) ) ;
#9974=ADVANCED_FACE ( 'NONE', ( #2653, #5780 ), #4837, .T. ) ;
#9976=CARTESIAN_POINT ( 'NONE',  ( 165.0000000000011369, 230.0000000000000853, 20.00000000000000000 ) ) ;
#9977=CARTESIAN_POINT ( 'NONE',  ( 74.62554477486000337, 42.37232431907235508, -24.41456952963950400 ) ) ;
#9979=ORIENTED_EDGE ( 'NONE', *, *, #5403, .F. ) ;
#9982=CARTESIAN_POINT ( 'NONE',  ( 70.10024745330821361, 14.62972355300540173, 26.66438925502398405 ) ) ;
#9985=CARTESIAN_POINT ( 'NONE',  ( 74.75803814165917061, 17.33402007532147593, 24.24257051231691307 ) ) ;
#9989=CARTESIAN_POINT ( 'NONE',  ( 71.40290628601371736, 44.01905189704749688, 23.11746242201492052 ) ) ;
#9991=DIRECTION ( 'NONE',  ( 0.000000000000000000, 0.000000000000000000, 1.000000000000000000 ) ) ;
#9993=DIRECTION ( 'NONE',  ( 1.224646799147352714E-16, 0.000000000000000000, -1.000000000000000000 ) ) ;
#9997=EDGE_CURVE ( 'NONE', #6378, #5388, #5028, .T. ) ;
#9998=EDGE_CURVE ( 'NONE', #3427, #6619, #8758, .T. ) ;
#9999=AXIS2_PLACEMENT_3D ( 'NONE', #11511, #4899, #5714 ) ;
#10008=CARTESIAN_POINT ( 'NONE',  ( 11.76612666199932811, 22.42800671064738793, 74.07172750083992696 ) ) ;
#10022=ADVANCED_BREP_SHAPE_REPRESENTATION ( '', ( #482, #1612 ), #10763 ) ;
#10023=DIRECTION ( 'NONE',  ( 0.000000000000000000, 0.000000000000000000, 1.000000000000000000 ) ) ;
#10025=CARTESIAN_POINT ( 'NONE',  ( 72.02465572632021917, 49.73463885619487002, -20.91766802171319029 ) ) ;
#10028=EDGE_CURVE ( 'NONE', #6205, #686, #3149, .T. ) ;
#10031=ORIENTED_EDGE ( 'NONE', *, *, #7015, .T. ) ;
#10041=CARTESIAN_POINT ( 'NONE',  ( 69.65391855624119444, 17.33976117116340632, 27.80917345409739383 ) ) ;
#10042=ADVANCED_FACE ( 'NONE', ( #7934 ), #2200, .T. ) ;
#10043=TOROIDAL_SURFACE ( 'NONE', #3478, 80.00000000000001421, 5.000000000000000000 ) ;
#10045=CARTESIAN_POINT ( 'NONE',  ( 74.40577577445179713, 18.24918190538344120, 24.69584740025122471 ) ) ;
#10049=CARTESIAN_POINT ( 'NONE',  ( 71.89872685388525042, 44.94434660361613254, 21.44363277848733063 ) ) ;
#10055=( BOUNDED_SURFACE ( )  B_SPLINE_SURFACE ( 3, 2, ( 
 ( #7750, #201, #9610 ),
 ( #7690, #1150, #1028 ),
 ( #75, #3892, #1087 ),
 ( #4890, #8678, #4370 ),
 ( #5080, #11811, #7122 ),
 ( #11871, #326, #3199 ),
 ( #2510, #6999, #573 ),
 ( #2378, #1331, #3322 ),
 ( #8856, #10920, #7061 ),
 ( #10985, #9796, #11931 ),
 ( #4250, #10858, #511 ),
 ( #3385, #8170, #5198 ),
 ( #6188, #383, #3255 ),
 ( #11993, #1269, #1514 ),
 ( #9036, #7983, #4132 ),
 ( #9982, #4311, #1452 ),
 ( #8916, #11049, #3449 ),
 ( #5141, #7249, #7923 ),
 ( #2321, #5257, #6128 ),
 ( #11741, #2449, #6252 ),
 ( #10041, #5319, #8105 ),
 ( #1387, #7185, #8977 ),
 ( #10798, #9918, #447 ),
 ( #8045, #6066, #9096 ),
 ( #2258, #9855, #4192 ),
 ( #9344, #12179, #3509 ) ),
 .UNSPECIFIED., .F., .F., .F. ) 
 B_SPLINE_SURFACE_WITH_KNOTS ( ( 4, 2, 2, 2, 2, 2, 2, 2, 2, 2, 2, 2, 4 ),
 ( 3, 3 ),
 ( 0.006933106248791173071, 0.008937828180681107321, 0.009940189146626074446, 0.01094255011257104157, 0.01294727204446097582, 0.01394963301040594295, 0.01495199397635090834, 0.01695671590824084085, 0.01795907687418580798, 0.01896143784013077510, 0.02096615977202070935, 0.02196852073796567648, 0.02297088170391064360 ),
 ( 0.000000000000000000, 1.000000000000000000 ),
 .UNSPECIFIED. ) 
 GEOMETRIC_REPRESENTATION_ITEM ( )  RATIONAL_B_SPLINE_SURFACE ( (
 ( 1.000000000000000000, 0.7071067811865475727, 1.000000000000000000),
 ( 1.000000000000000000, 0.7129067084832076961, 1.000000000000000000),
 ( 1.000000000000000000, 0.7190912265161553130, 1.000000000000000000),
 ( 1.000000000000000000, 0.7288225095607152593, 1.000000000000000000),
 ( 1.000000000000000000, 0.7321420440090222748, 1.000000000000000000),
 ( 1.000000000000000000, 0.7389120750275648408, 1.000000000000000000),
 ( 1.000000000000000000, 0.7423805904412675849, 1.000000000000000000),
 ( 1.000000000000000000, 0.7527643000948556207, 1.000000000000000000),
 ( 1.000000000000000000, 0.7596816647250912435, 1.000000000000000000),
 ( 1.000000000000000000, 0.7698812226851532436, 1.000000000000000000),
 ( 1.000000000000000000, 0.7732515396852113199, 1.000000000000000000),
 ( 1.000000000000000000, 0.7799012531313251895, 1.000000000000000000),
 ( 1.000000000000000000, 0.7831631659391242728, 1.000000000000000000),
 ( 1.000000000000000000, 0.7925626959609731736, 1.000000000000000000),
 ( 1.000000000000000000, 0.7983806636883555852, 1.000000000000000000),
 ( 1.000000000000000000, 0.8062586255457115936, 1.000000000000000000),
 ( 1.000000000000000000, 0.8087533637821711086, 1.000000000000000000),
 ( 1.000000000000000000, 0.8133656295006761461, 1.000000000000000000),
 ( 1.000000000000000000, 0.8154682471119866216, 1.000000000000000000),
 ( 1.000000000000000000, 0.8211473929488716239, 1.000000000000000000),
 ( 1.000000000000000000, 0.8241004955462830628, 1.000000000000000000),
 ( 1.000000000000000000, 0.8271253898583807995, 1.000000000000000000),
 ( 1.000000000000000000, 0.8278923858075547537, 1.000000000000000000),
 ( 1.000000000000000000, 0.8289041354387917115, 1.000000000000000000),
 ( 1.000000000000000000, 0.8291560334507810381, 1.000000000000000000),
 ( 1.000000000000000000, 0.8291561975888499525, 1.000000000000000000) ) ) 
 REPRESENTATION_ITEM ( '' )  SURFACE ( )  );
#10057=ORIENTED_EDGE ( 'NONE', *, *, #537, .F. ) ;
#10060=DIRECTION ( 'NONE',  ( 0.000000000000000000, 0.000000000000000000, 1.000000000000000000 ) ) ;
#10066=CARTESIAN_POINT ( 'NONE',  ( 13.80921887069453469, 29.53523948059399018, 73.71774192269633375 ) ) ;
#10067=CARTESIAN_POINT ( 'NONE',  ( 70.63701798748765270, 12.74415835139032716, -25.20839359252510548 ) ) ;
#10068=EDGE_CURVE ( 'NONE', #9474, #9777, #824, .T. ) ;
#10072=VECTOR ( 'NONE', #2092, 1000.000000000000000 ) ;
#10073=CYLINDRICAL_SURFACE ( 'NONE', #11596, 75.00000000000001421 ) ;
#10075=CARTESIAN_POINT ( 'NONE',  ( 77.12313347048127810, 44.96937891963703748, 20.63522338802521716 ) ) ;
#10076=ORIENTED_EDGE ( 'NONE', *, *, #2181, .F. ) ;
#10077=CYLINDRICAL_SURFACE ( 'NONE', #1693, 5.000000000000000888 ) ;
#10078=CARTESIAN_POINT ( 'NONE',  ( 77.29386075506074860, 15.00000000000009059, -20.32108226578737842 ) ) ;
#10084=ORIENTED_EDGE ( 'NONE', *, *, #3661, .F. ) ;
#10091=DIRECTION ( 'NONE',  ( 0.000000000000000000, 1.000000000000000000, 0.000000000000000000 ) ) ;
#10092=CARTESIAN_POINT ( 'NONE',  ( 77.45966692414833688, 10.00000000000009237, 20.00000000000000000 ) ) ;
#10097=DIRECTION ( 'NONE',  ( 0.000000000000000000, 0.000000000000000000, 1.000000000000000000 ) ) ;
#10098=ADVANCED_FACE ( 'NONE', ( #11575 ), #3029, .T. ) ;
#10101=CARTESIAN_POINT ( 'NONE',  ( 0.000000000000000000, 75.00000000000000000, 0.000000000000000000 ) ) ;
#10104=ORIENTED_EDGE ( 'NONE', *, *, #6008, .T. ) ;
#10106=CARTESIAN_POINT ( 'NONE',  ( 69.77609205918946600, 43.60216921429233139, 27.50116345873387758 ) ) ;
#10112=EDGE_CURVE ( 'NONE', #3229, #7980, #11699, .T. ) ;
#10119=DIRECTION ( 'NONE',  ( -0.7071067811865440200, 0.7071067811865510144, 0.000000000000000000 ) ) ;
#10122=CARTESIAN_POINT ( 'NONE',  ( -14.51674080820684054, 36.96222026613151002, 73.58288578104874489 ) ) ;
#10126=CARTESIAN_POINT ( 'NONE',  ( 9.184850993605150311E-15, 50.00000000000000000, 75.00000000000001421 ) ) ;
#10131=VECTOR ( 'NONE', #9967, 1000.000000000000000 ) ;
#10133=CARTESIAN_POINT ( 'NONE',  ( 0.000000000000000000, 50.00000000000000000, 0.000000000000000000 ) ) ;
#10136=CARTESIAN_POINT ( 'NONE',  ( 75.00000000000001421, 40.00000000000009237, 20.00000000000000000 ) ) ;
#10137=CARTESIAN_POINT ( 'NONE',  ( 76.05694877984106483, 15.60588465540594605, -22.40616324080664157 ) ) ;
#10147=EDGE_LOOP ( 'NONE', ( #6286, #819, #5554, #10968, #4140, #908 ) ) ;
#10148=DIRECTION ( 'NONE',  ( 0.000000000000000000, 0.000000000000000000, 1.000000000000000000 ) ) ;
#10163=CARTESIAN_POINT ( 'NONE',  ( 0.000000000000000000, 75.00000000000000000, 0.000000000000000000 ) ) ;
#10165=ORIENTED_EDGE ( 'NONE', *, *, #11767, .T. ) ;
#10170=DIRECTION ( 'NONE',  ( 1.000000000000000000, -0.000000000000000000, 0.000000000000000000 ) ) ;
#10171=CARTESIAN_POINT ( 'NONE',  ( 71.95778018440438473, 49.67323215106386414, 21.14640536576772689 ) ) ;
#10188=DIRECTION ( 'NONE',  ( 0.000000000000000000, 0.000000000000000000, 1.000000000000000000 ) ) ;
#10194=AXIS2_PLACEMENT_3D ( 'NONE', #9617, #210, #11386 ) ;
#10206=EDGE_CURVE ( 'NONE', #9199, #5882, #7392, .T. ) ;
#10207=ORIENTED_EDGE ( 'NONE', *, *, #9787, .T. ) ;
#10220=DIRECTION ( 'NONE',  ( -1.000000000000000000, 0.000000000000000000, -0.000000000000000000 ) ) ;
#10221=CIRCLE ( 'NONE', #4856, 70.00000000000001421 ) ;
#10226=ADVANCED_FACE ( 'NONE', ( #841 ), #7388, .F. ) ;
#10227=DIRECTION ( 'NONE',  ( 0.000000000000000000, 0.000000000000000000, 1.000000000000000000 ) ) ;
#10231=CARTESIAN_POINT ( 'NONE',  ( 0.000000000000000000, 50.00000000000008527, 0.000000000000000000 ) ) ;
#10236=CARTESIAN_POINT ( 'NONE',  ( 0.000000000000000000, 106.9570738953063085, 0.000000000000000000 ) ) ;
#10252=CARTESIAN_POINT ( 'NONE',  ( -10.60456947870001976, 41.68965759107759794, 74.24767693116807266 ) ) ;
#10253=DIRECTION ( 'NONE',  ( 0.000000000000000000, -0.000000000000000000, 1.000000000000000000 ) ) ;
#10268=AXIS2_PLACEMENT_3D ( 'NONE', #3276, #4090, #10632 ) ;
#10273=CIRCLE ( 'NONE', #327, 10.00000000000000178 ) ;
#10279=VECTOR ( 'NONE', #5823, 1000.000000000000000 ) ;
#10286=LINE ( 'NONE', #1815, #10977 ) ;
#10288=ADVANCED_FACE ( 'NONE', ( #3638 ), #7447, .T. ) ;
#10292=ORIENTED_EDGE ( 'NONE', *, *, #609, .F. ) ;
#10294=CARTESIAN_POINT ( 'NONE',  ( -16.05603493625720546, 27.92803657533481498, 73.26122286506979719 ) ) ;
#10297=CARTESIAN_POINT ( 'NONE',  ( -30.00000000000004263, 65.00000000000000000, 63.24555320336758513 ) ) ;
#10299=CARTESIAN_POINT ( 'NONE',  ( 0.000000000000000000, -10.00000000000000000, 0.000000000000000000 ) ) ;
#10300=DIRECTION ( 'NONE',  ( 0.000000000000000000, 0.000000000000000000, -1.000000000000000000 ) ) ;
#10303=ORIENTED_EDGE ( 'NONE', *, *, #3630, .T. ) ;
#10308=CARTESIAN_POINT ( 'NONE',  ( -16.19078112930547064, 30.00000000000008882, 73.23154106273422315 ) ) ;
#10311=CARTESIAN_POINT ( 'NONE',  ( 145.0000000000011369, 225.0000000000000853, 25.00000000000000000 ) ) ;
#10313=CARTESIAN_POINT ( 'NONE',  ( -9.777035353469207379, 42.31031047869488049, 74.36117268575515027 ) ) ;
#10317=CARTESIAN_POINT ( 'NONE',  ( 3.202269328900650969, 15.65019529770482443, 74.93294739197928322 ) ) ;
#10329=ORIENTED_EDGE ( 'NONE', *, *, #1622, .F. ) ;
#10333=AXIS2_PLACEMENT_3D ( 'NONE', #12098, #5424, #11219 ) ;
#10334=LINE ( 'NONE', #12348, #8207 ) ;
#10336=CARTESIAN_POINT ( 'NONE',  ( 0.000000000000000000, 109.0000000000000000, 3.399999999999999911 ) ) ;
#10347=EDGE_CURVE ( 'NONE', #8527, #44, #9791, .T. ) ;
#10348=DIRECTION ( 'NONE',  ( 0.000000000000000000, 1.000000000000000000, 0.000000000000000000 ) ) ;
#10352=EDGE_CURVE ( 'NONE', #737, #10899, #8959, .T. ) ;
#10359=AXIS2_PLACEMENT_3D ( 'NONE', #10810, #400, #7880 ) ;
#10368=CIRCLE ( 'NONE', #9568, 5.000000000000004441 ) ;
#10372=AXIS2_PLACEMENT_3D ( 'NONE', #4182, #10850, #2313 ) ;
#10376=DIRECTION ( 'NONE',  ( 0.000000000000000000, 1.000000000000000000, 0.000000000000000000 ) ) ;
#10378=CARTESIAN_POINT ( 'NONE',  ( 125.0000000000009663, 42.92893218813456713, -20.00000000000000000 ) ) ;
#10385=CARTESIAN_POINT ( 'NONE',  ( 69.52686081653675387, 40.33415354502060524, -28.12499999996316546 ) ) ;
#10389=DIRECTION ( 'NONE',  ( -3.469446951953613203E-16, 0.000000000000000000, -1.000000000000000000 ) ) ;
#10391=VERTEX_POINT ( 'NONE', #261 ) ;
#10395=EDGE_LOOP ( 'NONE', ( #2676, #8901, #3391, #8601 ) ) ;
#10401=ORIENTED_EDGE ( 'NONE', *, *, #5151, .F. ) ;
#10403=CARTESIAN_POINT ( 'NONE',  ( 150.0000000000010516, 15.00000000000008704, -22.92893218813451384 ) ) ;
#10417=CARTESIAN_POINT ( 'NONE',  ( 69.65097664248530407, 42.56552300069557049, 27.81636932325739409 ) ) ;
#10420=CARTESIAN_POINT ( 'NONE',  ( 72.32585155008058564, 45.16148467125184851, 19.87486525338015042 ) ) ;
#10421=CIRCLE ( 'NONE', #5060, 4.999999999999996447 ) ;
#10433=CIRCLE ( 'NONE', #2873, 80.00000000000001421 ) ;
#10444=( LENGTH_UNIT ( ) NAMED_UNIT ( * ) SI_UNIT ( .MILLI., .METRE. ) );
#10446=CARTESIAN_POINT ( 'NONE',  ( 76.56943592554333122, 44.74351910189555070, -21.58906638518922705 ) ) ;
#10447=VECTOR ( 'NONE', #5804, 1000.000000000000114 ) ;
#10448=FILL_AREA_STYLE_COLOUR ( '', #719 ) ;
#10449=ORIENTED_EDGE ( 'NONE', *, *, #4668, .T. ) ;
#10453=CARTESIAN_POINT ( 'NONE',  ( 76.19870213673728188, 15.49246197672877834, -22.18755841417196351 ) ) ;
#10455=EDGE_CURVE ( 'NONE', #3552, #9442, #11683, .T. ) ;
#10456=DIRECTION ( 'NONE',  ( -0.000000000000000000, -1.000000000000000000, -0.000000000000000000 ) ) ;
#10469=ORIENTED_EDGE ( 'NONE', *, *, #2441, .T. ) ;
#10474=ORIENTED_EDGE ( 'NONE', *, *, #2540, .T. ) ;
#10482=EDGE_LOOP ( 'NONE', ( #3939, #10474, #6565, #3112 ) ) ;
#10494=EDGE_CURVE ( 'NONE', #9831, #7679, #5005, .T. ) ;
#10496=ORIENTED_EDGE ( 'NONE', *, *, #5403, .T. ) ;
#10497=EDGE_LOOP ( 'NONE', ( #10329, #9327, #3096, #1019 ) ) ;
#10498=CARTESIAN_POINT ( 'NONE',  ( 0.000000000000000000, 5.000000000000129674, 0.000000000000000000 ) ) ;
#10504=CARTESIAN_POINT ( 'NONE',  ( 0.000000000000000000, 115.0000000000000000, 0.000000000000000000 ) ) ;
#10506=VERTEX_POINT ( 'NONE', #8041 ) ;
#10509=CARTESIAN_POINT ( 'NONE',  ( 71.17928254424892032, 43.30619889802275679, -23.82724229592531273 ) ) ;
#10525=CARTESIAN_POINT ( 'NONE',  ( 74.19368986856427739, 40.71666413485492342, 24.96097029013992241 ) ) ;
#10528=DIRECTION ( 'NONE',  ( 0.000000000000000000, 0.000000000000000000, -1.000000000000000000 ) ) ;
#10533=VERTEX_POINT ( 'NONE', #1327 ) ;
#10537=AXIS2_PLACEMENT_3D ( 'NONE', #3102, #5913, #4041 ) ;
#10548=DIRECTION ( 'NONE',  ( -0.000000000000000000, 1.000000000000000000, -0.000000000000000000 ) ) ;
#10549=CARTESIAN_POINT ( 'NONE',  ( 117.9289321881355193, 40.00000000000009237, 20.00000000000000000 ) ) ;
#10554=( BOUNDED_SURFACE ( )  B_SPLINE_SURFACE ( 3, 2, ( 
 ( #1519, #8049, #9100 ),
 ( #11814, #3325, #6945 ),
 ( #1455, #3257, #7125 ),
 ( #329, #7065, #2324 ),
 ( #6131, #1391, #10923 ),
 ( #2381, #923, #10446 ),
 ( #9626, #3204, #2780 ),
 ( #1107, #5722, #7004 ),
 ( #5784, #7927, #11520 ),
 ( #2039, #8695, #9861 ),
 ( #2909, #6772, #1913 ),
 ( #5144, #11395, #7708 ),
 ( #1974, #4911, #4198 ),
 ( #2972, #4843, #9566 ),
 ( #1847, #2847, #10571 ),
 ( #5842, #10509, #94 ),
 ( #10801, #983, #8630 ),
 ( #1042, #5660, #3968 ),
 ( #8920, #390, #4715 ),
 ( #9439, #4776, #11750 ),
 ( #6648, #6587, #8567 ),
 ( #8507, #7645, #6071 ),
 ( #3911, #157, #31 ),
 ( #2261, #1336, #11332 ),
 ( #10385, #12330, #9500 ),
 ( #3778, #6713, #7581 ) ),
 .UNSPECIFIED., .F., .F., .F. ) 
 B_SPLINE_SURFACE_WITH_KNOTS ( ( 4, 2, 2, 2, 2, 2, 2, 2, 2, 2, 2, 2, 4 ),
 ( 3, 3 ),
 ( 0.006933106248791174805, 0.008937828180681107321, 0.009940189146626074446, 0.01094255011257104157, 0.01294727204446097409, 0.01394963301040593948, 0.01495199397635090660, 0.01695671590824084085, 0.01795907687418580798, 0.01896143784013077510, 0.02096615977202070935, 0.02196852073796567301, 0.02297088170391064013 ),
 ( 0.000000000000000000, 1.000000000000000000 ),
 .UNSPECIFIED. ) 
 GEOMETRIC_REPRESENTATION_ITEM ( )  RATIONAL_B_SPLINE_SURFACE ( (
 ( 1.000000000000000000, 0.7071067811865475727, 1.000000000000000000),
 ( 1.000000000000000000, 0.7129067084832356738, 1.000000000000000000),
 ( 1.000000000000000000, 0.7190912265161183425, 1.000000000000000000),
 ( 1.000000000000000000, 0.7288225095607339110, 1.000000000000000000),
 ( 1.000000000000000000, 0.7321420440090409265, 1.000000000000000000),
 ( 1.000000000000000000, 0.7389120750275461891, 1.000000000000000000),
 ( 1.000000000000000000, 0.7423805904413234291, 1.000000000000000000),
 ( 1.000000000000000000, 0.7527643000947431551, 1.000000000000000000),
 ( 1.000000000000000000, 0.7596816647252027099, 1.000000000000000000),
 ( 1.000000000000000000, 0.7698812226850976215, 1.000000000000000000),
 ( 1.000000000000000000, 0.7732515396852110978, 1.000000000000000000),
 ( 1.000000000000000000, 0.7799012531313249674, 1.000000000000000000),
 ( 1.000000000000000000, 0.7831631659391801170, 1.000000000000000000),
 ( 1.000000000000000000, 0.7925626959608614852, 1.000000000000000000),
 ( 1.000000000000000000, 0.7983806636883183927, 1.000000000000000000),
 ( 1.000000000000000000, 0.8062586255457302453, 1.000000000000000000),
 ( 1.000000000000000000, 0.8087533637821522348, 1.000000000000000000),
 ( 1.000000000000000000, 0.8133656295006947978, 1.000000000000000000),
 ( 1.000000000000000000, 0.8154682471119685250, 1.000000000000000000),
 ( 1.000000000000000000, 0.8211473929489091494, 1.000000000000000000),
 ( 1.000000000000000000, 0.8241004955462456483, 1.000000000000000000),
 ( 1.000000000000000000, 0.8271253898583996733, 1.000000000000000000),
 ( 1.000000000000000000, 0.8278923858075547537, 1.000000000000000000),
 ( 1.000000000000000000, 0.8289041354387917115, 1.000000000000000000),
 ( 1.000000000000000000, 0.8291560334507813712, 1.000000000000000000),
 ( 1.000000000000000000, 0.8291561975888499525, 1.000000000000000000) ) ) 
 REPRESENTATION_ITEM ( '' )  SURFACE ( )  );
#10559=CARTESIAN_POINT ( 'NONE',  ( 8.122470672675945025, 41.76773423473973423, 74.55981757952413602 ) ) ;
#10560=ORIENTED_EDGE ( 'NONE', *, *, #5125, .T. ) ;
#10570=ADVANCED_FACE ( 'NONE', ( #7979 ), #11807, .T. ) ;
#10571=CARTESIAN_POINT ( 'NONE',  ( 74.98307306353127899, 43.09120835303954777, -23.94359236839000360 ) ) ;
#10572=PRESENTATION_STYLE_ASSIGNMENT (( #8696 ) ) ;
#10573=AXIS2_PLACEMENT_3D ( 'NONE', #9959, #3431, #364 ) ;
#10575=B_SPLINE_CURVE_WITH_KNOTS ( 'NONE', 3,
 ( #4897, #9736, #2961, #1032, #208, #5954, #3900, #4081, #4958, #7874, #4019, #6758, #7633, #6948, #10559, #5086, #2027, #11447, #1217, #5021, #2898, #7818, #6824, #5894 ),
 .UNSPECIFIED., .F., .F.,
 ( 4, 2, 2, 2, 2, 2, 2, 2, 2, 2, 2, 4 ),
 ( 0.02230690517119256200, 0.02509601044920642052, 0.02788511572722027904, 0.02927966836622719615, 0.03067422100523411674, 0.03346332628324795444, 0.03485787892225486462, 0.03625243156126176786, 0.03904153683927557433, 0.04043608947828247757, 0.04183064211728938775, 0.04461974739530318729 ),
 .UNSPECIFIED. ) ;
#10576=CARTESIAN_POINT ( 'NONE',  ( 143.5355339059338462, 61.46446609406724804, -25.00000000000000000 ) ) ;
#10578=CARTESIAN_POINT ( 'NONE',  ( 71.31012073600892620, 16.24668676079221896, -23.41524959671153638 ) ) ;
#10589=CARTESIAN_POINT ( 'NONE',  ( 76.05694877984102220, 44.39411534459425468, 22.40616324080664157 ) ) ;
#10591=APPLICATION_CONTEXT ( 'automotive_design' ) ;
#10597=FACE_OUTER_BOUND ( 'NONE', #1717, .T. ) ;
#10609=DIRECTION ( 'NONE',  ( 0.000000000000000000, 1.000000000000000000, 0.000000000000000000 ) ) ;
#10610=EDGE_CURVE ( 'NONE', #686, #10506, #6183, .T. ) ;
#10619=VERTEX_POINT ( 'NONE', #6434 ) ;
#10620=AXIS2_PLACEMENT_3D ( 'NONE', #4216, #11894, #11830 ) ;
#10631=ORIENTED_EDGE ( 'NONE', *, *, #11728, .F. ) ;
#10632=DIRECTION ( 'NONE',  ( -1.000000000000000000, 0.000000000000000000, 0.000000000000000000 ) ) ;
#10638=CARTESIAN_POINT ( 'NONE',  ( 70.30108951986159127, 13.82498561756345445, -26.13045860990803249 ) ) ;
#10642=EDGE_CURVE ( 'NONE', #6005, #10667, #6499, .T. ) ;
#10645=EDGE_CURVE ( 'NONE', #6005, #11474, #10368, .T. ) ;
#10652=LINE ( 'NONE', #8650, #9834 ) ;
#10659=ORIENTED_EDGE ( 'NONE', *, *, #11441, .T. ) ;
#10663=VECTOR ( 'NONE', #9848, 1000.000000000000114 ) ;
#10666=FACE_OUTER_BOUND ( 'NONE', #8926, .T. ) ;
#10667=VERTEX_POINT ( 'NONE', #8412 ) ;
#10668=AXIS2_PLACEMENT_3D ( 'NONE', #5421, #3604, #2785 ) ;
#10669=DIRECTION ( 'NONE',  ( 1.000000000000000000, -0.000000000000000000, 0.000000000000000000 ) ) ;
#10675=CARTESIAN_POINT ( 'NONE',  ( 74.40577577445179713, 41.75081809461674709, -24.69584740025122471 ) ) ;
#10678=CARTESIAN_POINT ( 'NONE',  ( 170.0000000000011369, 225.0000000000000853, -19.99999999999999645 ) ) ;
#10681=ORIENTED_EDGE ( 'NONE', *, *, #3331, .F. ) ;
#10683=CARTESIAN_POINT ( 'NONE',  ( 170.0000000000011369, 35.00000000000004974, 20.00000000000000000 ) ) ;
#10689=LINE ( 'NONE', #8690, #5512 ) ;
#10697=CARTESIAN_POINT ( 'NONE',  ( 145.0000000000011369, 225.0000000000000853, 20.00000000000000000 ) ) ;
#10698=CARTESIAN_POINT ( 'NONE',  ( 76.75496552995652166, 15.16338392435726945, -21.27808286176472308 ) ) ;
#10699=DIRECTION ( 'NONE',  ( 0.000000000000000000, 0.000000000000000000, -1.000000000000000000 ) ) ;
#10703=EDGE_CURVE ( 'NONE', #1747, #4020, #10286, .T. ) ;
#10711=ADVANCED_FACE ( 'NONE', ( #1870 ), #2743, .T. ) ;
#10714=ORIENTED_EDGE ( 'NONE', *, *, #9128, .F. ) ;
#10725=DIRECTION ( 'NONE',  ( 0.000000000000000000, -0.000000000000000000, 1.000000000000000000 ) ) ;
#10735=PLANE ( 'NONE',  #6768 ) ;
#10740=VERTEX_POINT ( 'NONE', #305 ) ;
#10742=VERTEX_POINT ( 'NONE', #8837 ) ;
#10745=CARTESIAN_POINT ( 'NONE',  ( 0.000000000000000000, 63.00000000000000000, -57.08203932499371547 ) ) ;
#10747=CARTESIAN_POINT ( 'NONE',  ( 2.020667218593133416E-14, 63.00000000000000000, 70.00000000000000000 ) ) ;
#10750=DIRECTION ( 'NONE',  ( -0.000000000000000000, 1.000000000000000000, -0.000000000000000000 ) ) ;
#10751=AXIS2_PLACEMENT_3D ( 'NONE', #9567, #3846, #9441 ) ;
#10752=CARTESIAN_POINT ( 'NONE',  ( 0.000000000000000000, 65.00000000000000000, -57.08203932499371547 ) ) ;
#10757=CYLINDRICAL_SURFACE ( 'NONE', #3306, 75.00000000000001421 ) ;
#10760=CARTESIAN_POINT ( 'NONE',  ( 0.000000000000000000, 20.00000000000009237, 20.00000000000000000 ) ) ;
#10763=( GEOMETRIC_REPRESENTATION_CONTEXT ( 3 ) GLOBAL_UNCERTAINTY_ASSIGNED_CONTEXT ( ( #2397 ) ) GLOBAL_UNIT_ASSIGNED_CONTEXT ( ( #218, #6833, #2100 ) ) REPRESENTATION_CONTEXT ( 'NONE', 'WORKASPACE' ) );
#10768=VERTEX_POINT ( 'NONE', #6922 ) ;
#10777=EDGE_LOOP ( 'NONE', ( #6160, #7870, #9055, #11319 ) ) ;
#10786=CARTESIAN_POINT ( 'NONE',  ( -11.74466661846254034, 19.32863853742761862, 74.07568943800757211 ) ) ;
#10790=VERTEX_POINT ( 'NONE', #9710 ) ;
#10792=CARTESIAN_POINT ( 'NONE',  ( 74.16198487095665826, 0.000000000000000000, -25.00000000000000000 ) ) ;
#10798=CARTESIAN_POINT ( 'NONE',  ( 69.55864520994451539, 18.66433107818797055, 28.04631938806005564 ) ) ;
#10801=CARTESIAN_POINT ( 'NONE',  ( 70.03799559100568217, 45.08708461952503654, -26.82731484558848578 ) ) ;
#10804=CARTESIAN_POINT ( 'NONE',  ( 71.13616097333213872, 43.15315690759868517, 23.96252879557600934 ) ) ;
#10810=CARTESIAN_POINT ( 'NONE',  ( 1.734723475976807094E-14, 63.00000000000000000, 57.08203932499370836 ) ) ;
#10814=VERTEX_POINT ( 'NONE', #8780 ) ;
#10815=CIRCLE ( 'NONE', #10620, 5.000000000000004441 ) ;
#10818=DIRECTION ( 'NONE',  ( 0.000000000000000000, 0.000000000000000000, 1.000000000000000000 ) ) ;
#10830=ORIENTED_EDGE ( 'NONE', *, *, #7376, .T. ) ;
#10835=FACE_OUTER_BOUND ( 'NONE', #9319, .T. ) ;
#10838=FACE_OUTER_BOUND ( 'NONE', #8277, .T. ) ;
#10841=CARTESIAN_POINT ( 'NONE',  ( 70.01409082250448535, 44.97240956491599917, -26.88960057466319498 ) ) ;
#10850=DIRECTION ( 'NONE',  ( 0.000000000000000000, -0.000000000000000000, 1.000000000000000000 ) ) ;
#10851=DIRECTION ( 'NONE',  ( -0.000000000000000000, 1.000000000000000000, -0.000000000000000000 ) ) ;
#10855=DIRECTION ( 'NONE',  ( 0.000000000000000000, 0.000000000000000000, 1.000000000000000000 ) ) ;
#10858=CARTESIAN_POINT ( 'NONE',  ( 71.69656859387025349, 15.34954140224283847, 22.14271594285881051 ) ) ;
#10859=VECTOR ( 'NONE', #2947, 1000.000000000000000 ) ;
#10860=AXIS2_PLACEMENT_3D ( 'NONE', #11539, #5862, #3053 ) ;
#10866=CARTESIAN_POINT ( 'NONE',  ( 71.05921646411503900, 42.81507391128047857, 24.19824146092189920 ) ) ;
#10871=CARTESIAN_POINT ( 'NONE',  ( 140.0000000000011369, 230.0000000000000853, 20.00000000000000000 ) ) ;
#10872=CIRCLE ( 'NONE', #10268, 5.000000000000004441 ) ;
#10892=ADVANCED_FACE ( 'NONE', ( #10597 ), #5177, .T. ) ;
#10898=CARTESIAN_POINT ( 'NONE',  ( 75.04216158314673635, 16.80959580454246094, -23.86402193374160774 ) ) ;
#10899=VERTEX_POINT ( 'NONE', #5238 ) ;
#10903=CARTESIAN_POINT ( 'NONE',  ( 71.40042903152233578, 48.95734231283034177, -22.96380533506442845 ) ) ;
#10904=AXIS2_PLACEMENT_3D ( 'NONE', #1563, #10148, #4356 ) ;
#10910=CARTESIAN_POINT ( 'NONE',  ( 0.000000000000000000, 10.00000000000017586, 0.000000000000000000 ) ) ;
#10912=ORIENTED_EDGE ( 'NONE', *, *, #9960, .F. ) ;
#10920=CARTESIAN_POINT ( 'NONE',  ( 71.89703483712752075, 15.05775874217476940, 21.44956398269973619 ) ) ;
#10923=CARTESIAN_POINT ( 'NONE',  ( 76.75412411316109740, 44.83621509884553546, -21.27950340534319906 ) ) ;
#10926=DIRECTION ( 'NONE',  ( -0.7071067811865454633, 0.7071067811865495711, 0.000000000000000000 ) ) ;
#10927=CARTESIAN_POINT ( 'NONE',  ( 74.30294665491157957, 41.32313156420044464, 24.82467190422428516 ) ) ;
#10937=ORIENTED_EDGE ( 'NONE', *, *, #9205, .T. ) ;
#10939=CARTESIAN_POINT ( 'NONE',  ( 8.572527594031474570E-15, -5.000000000000000000, -70.00000000000001421 ) ) ;
#10943=DIRECTION ( 'NONE',  ( 0.000000000000000000, 0.000000000000000000, -1.000000000000000000 ) ) ;
#10956=ORIENTED_EDGE ( 'NONE', *, *, #10494, .T. ) ;
#10961=LINE ( 'NONE', #2423, #5856 ) ;
#10965=VERTEX_POINT ( 'NONE', #11027 ) ;
#10966=CARTESIAN_POINT ( 'NONE',  ( 69.57537924859245493, 41.62899728819233758, -28.00483409347995689 ) ) ;
#10968=ORIENTED_EDGE ( 'NONE', *, *, #8805, .F. ) ;
#10976=DIRECTION ( 'NONE',  ( -1.000000000000000000, -0.000000000000000000, -0.000000000000000000 ) ) ;
#10977=VECTOR ( 'NONE', #11235, 1000.000000000000000 ) ;
#10985=CARTESIAN_POINT ( 'NONE',  ( 71.00573438501008638, 11.81969099518210520, 24.15070487907408037 ) ) ;
#10988=CARTESIAN_POINT ( 'NONE',  ( 77.12362621866023460, 15.03061249690207291, 20.63427607811778230 ) ) ;
#10991=EDGE_CURVE ( 'NONE', #298, #2246, #1388, .T. ) ;
#10994=CARTESIAN_POINT ( 'NONE',  ( 75.64998878962165918, 43.99497189443935952, 23.01105902605777231 ) ) ;
#10996=SPHERICAL_SURFACE ( 'NONE', #5502, 5.000000000000000000 ) ;
#11000=ORIENTED_EDGE ( 'NONE', *, *, #6395, .F. ) ;
#11005=CARTESIAN_POINT ( 'NONE',  ( 165.0000000000011369, 225.0000000000000853, -19.99999999999999645 ) ) ;
#11009=CARTESIAN_POINT ( 'NONE',  ( 121.4644660940682428, 46.46446609406732620, 20.00000000000000000 ) ) ;
#11016=B_SPLINE_CURVE_WITH_KNOTS ( 'NONE', 3,
 ( #3884, #5818, #7621, #7806, #5938, #6933, #2882, #11429, #9603, #6690, #1017, #4818, #8606, #5132, #11803, #11986, #3443, #2191, #7913, #3246, #7239, #9089, #5999, #6059 ),
 .UNSPECIFIED., .F., .F.,
 ( 4, 2, 2, 2, 2, 2, 2, 2, 2, 2, 2, 4 ),
 ( 0.000000000000000000, 0.0009796746052621193267, 0.001959349210524238653, 0.003918698421048477307, 0.004898373026310590128, 0.005878047631572703817, 0.007837396842096925123, 0.009796746052621145562, 0.01175609526314536774, 0.01273576986840747882, 0.01371544447366958817, 0.01567479368419381902 ),
 .UNSPECIFIED. ) ;
#11017=ORIENTED_EDGE ( 'NONE', *, *, #2280, .T. ) ;
#11022=CARTESIAN_POINT ( 'NONE',  ( 76.77294714683046095, 15.14884821498869094, -21.25082451143516948 ) ) ;
#11023=ORIENTED_EDGE ( 'NONE', *, *, #5030, .T. ) ;
#11027=CARTESIAN_POINT ( 'NONE',  ( 117.9289321881355193, 45.00000000000008527, -20.00000000000000000 ) ) ;
#11029=CARTESIAN_POINT ( 'NONE',  ( 145.0000000000011369, 67.07106781186550393, 25.00000000000000000 ) ) ;
#11033=ORIENTED_EDGE ( 'NONE', *, *, #7673, .F. ) ;
#11037=VERTEX_POINT ( 'NONE', #6112 ) ;
#11041=EDGE_CURVE ( 'NONE', #11684, #2560, #12339, .T. ) ;
#11048=ADVANCED_FACE ( 'NONE', ( #10838 ), #587, .T. ) ;
#11049=CARTESIAN_POINT ( 'NONE',  ( 71.13813068160065711, 16.85611227734841933, 23.95492789737738804 ) ) ;
#11050=AXIS2_PLACEMENT_3D ( 'NONE', #1245, #1306, #3296 ) ;
#11056=DIRECTION ( 'NONE',  ( 0.000000000000000000, 0.000000000000000000, 1.000000000000000000 ) ) ;
#11057=ORIENTED_EDGE ( 'NONE', *, *, #10206, .F. ) ;
#11059=CARTESIAN_POINT ( 'NONE',  ( 75.74050859682202486, 44.09128781609246772, 22.87883167916283256 ) ) ;
#11060=ORIENTED_EDGE ( 'NONE', *, *, #2955, .F. ) ;
#11066=ORIENTED_EDGE ( 'NONE', *, *, #8599, .F. ) ;
#11068=AXIS2_PLACEMENT_3D ( 'NONE', #7567, #5582, #11375 ) ;
#11070=CONICAL_SURFACE ( 'NONE', #309, 75.00000000000001421, 0.7853981633974427279 ) ;
#11078=CARTESIAN_POINT ( 'NONE',  ( -16.08467657231584624, 32.05922307041088004, 73.25523918613529872 ) ) ;
#11079=CARTESIAN_POINT ( 'NONE',  ( 74.16198487095664404, 20.00000000000009237, -29.99999999999999645 ) ) ;
#11082=LINE ( 'NONE', #8322, #8947 ) ;
#11086=CARTESIAN_POINT ( 'NONE',  ( 1.857738790484679381, 15.28369354803722402, 74.98235353336227149 ) ) ;
#11094=AXIS2_PLACEMENT_3D ( 'NONE', #9806, #1283, #5090 ) ;
#11101=PLANE ( 'NONE',  #2052 ) ;
#11129=ORIENTED_EDGE ( 'NONE', *, *, #982, .F. ) ;
#11130=DIRECTION ( 'NONE',  ( -1.000000000000000000, 0.000000000000000000, 0.000000000000000000 ) ) ;
#11136=CARTESIAN_POINT ( 'NONE',  ( -16.19078112930547775, 31.03558258355681687, 73.23154106273423736 ) ) ;
#11138=CARTESIAN_POINT ( 'NONE',  ( 70.40913241174638415, 13.44666843646714405, -25.83788073351890802 ) ) ;
#11142=CIRCLE ( 'NONE', #5776, 4.999999999999997335 ) ;
#11149=CARTESIAN_POINT ( 'NONE',  ( 74.42783152987426831, 18.19891539281256598, -24.66728717810469362 ) ) ;
#11153=DIRECTION ( 'NONE',  ( -0.7071067811865455743, 0.7071067811865495711, 0.000000000000000000 ) ) ;
#11160=ORIENTED_EDGE ( 'NONE', *, *, #9499, .F. ) ;
#11161=CARTESIAN_POINT ( 'NONE',  ( 0.000000000000000000, 50.00000000000000000, -75.00000000000001421 ) ) ;
#11165=FACE_OUTER_BOUND ( 'NONE', #10482, .T. ) ;
#11166=ORIENTED_EDGE ( 'NONE', *, *, #3756, .T. ) ;
#11172=COLOUR_RGB ( '', 0.66274510, 0.83137255, 0.94901961) ;
#11173=EDGE_LOOP ( 'NONE', ( #7871, #3298, #9097, #9362 ) ) ;
#11175=CARTESIAN_POINT ( 'NONE',  ( 165.0000000000011369, 225.0000000000000853, 25.00000000000000000 ) ) ;
#11180=CARTESIAN_POINT ( 'NONE',  ( 71.39985347493268364, 48.95609667407049415, 22.96547907468804084 ) ) ;
#11183=DIRECTION ( 'NONE',  ( 0.000000000000000000, 1.000000000000000000, 0.000000000000000000 ) ) ;
#11188=AXIS2_PLACEMENT_3D ( 'NONE', #5160, #4092, #1290 ) ;
#11191=VECTOR ( 'NONE', #11485, 1000.000000000000000 ) ;
#11193=ORIENTED_EDGE ( 'NONE', *, *, #5852, .T. ) ;
#11196=CARTESIAN_POINT ( 'NONE',  ( 0.000000000000000000, 109.0000000000000000, 0.000000000000000000 ) ) ;
#11200=EDGE_CURVE ( 'NONE', #5052, #11037, #4571, .T. ) ;
#11208=CIRCLE ( 'NONE', #7422, 3.399999999999999911 ) ;
#11210=ORIENTED_EDGE ( 'NONE', *, *, #6412, .T. ) ;
#11211=ADVANCED_FACE ( 'NONE', ( #3548 ), #9202, .F. ) ;
#11215=CARTESIAN_POINT ( 'NONE',  ( 0.000000000000000000, 115.0000000000000000, 9.999999999999998224 ) ) ;
#11219=DIRECTION ( 'NONE',  ( 0.000000000000000000, 0.000000000000000000, 1.000000000000000000 ) ) ;
#11233=FACE_OUTER_BOUND ( 'NONE', #11880, .T. ) ;
#11235=DIRECTION ( 'NONE',  ( -0.000000000000000000, -1.000000000000000000, -0.000000000000000000 ) ) ;
#11246=CARTESIAN_POINT ( 'NONE',  ( 69.89773400907223788, 44.39854272105920785, 27.19132888315843033 ) ) ;
#11259=ORIENTED_EDGE ( 'NONE', *, *, #376, .F. ) ;
#11262=ADVANCED_FACE ( 'NONE', ( #7775 ), #8576, .T. ) ;
#11267=CIRCLE ( 'NONE', #5292, 3.399999999999999911 ) ;
#11270=CARTESIAN_POINT ( 'NONE',  ( -7.093000575290183463, 43.82875375259622075, 74.67028158002766247 ) ) ;
#11277=VECTOR ( 'NONE', #10528, 1000.000000000000000 ) ;
#11279=EDGE_LOOP ( 'NONE', ( #9859, #9027, #3546, #3330 ) ) ;
#11288=VERTEX_POINT ( 'NONE', #9698 ) ;
#11293=EDGE_LOOP ( 'NONE', ( #10207, #8811, #7757, #177 ) ) ;
#11296=ORIENTED_EDGE ( 'NONE', *, *, #11200, .F. ) ;
#11306=CARTESIAN_POINT ( 'NONE',  ( 165.0000000000011369, 35.00000000000004974, -25.00000000000000000 ) ) ;
#11307=CARTESIAN_POINT ( 'NONE',  ( -15.13458840481166590, 24.44672303875686481, 73.45739858620734708 ) ) ;
#11309=CARTESIAN_POINT ( 'NONE',  ( 0.000000000000000000, 115.0000000000000000, 3.399999999999999911 ) ) ;
#11310=CARTESIAN_POINT ( 'NONE',  ( 72.61843774138908714, 45.00000000000009948, 18.75000000000000711 ) ) ;
#11311=ORIENTED_EDGE ( 'NONE', *, *, #10068, .F. ) ;
#11319=ORIENTED_EDGE ( 'NONE', *, *, #8599, .T. ) ;
#11327=CONICAL_SURFACE ( 'NONE', #3748, 3.399999999999999911, 1.029744258676658974 ) ;
#11328=FACE_OUTER_BOUND ( 'NONE', #1390, .T. ) ;
#11330=ORIENTED_EDGE ( 'NONE', *, *, #12207, .F. ) ;
#11332=CARTESIAN_POINT ( 'NONE',  ( 74.16874958671132845, 40.33405953496801999, -24.99164682819347760 ) ) ;
#11336=FACE_OUTER_BOUND ( 'NONE', #2945, .T. ) ;
#11337=CARTESIAN_POINT ( 'NONE',  ( 70.88237045016090576, 18.32754774912132234, -24.73035864412310758 ) ) ;
#11339=DIRECTION ( 'NONE',  ( -1.000000000000000000, 0.000000000000000000, 0.000000000000000000 ) ) ;
#11343=AXIS2_PLACEMENT_3D ( 'NONE', #1013, #3003, #3064 ) ;
#11348=CIRCLE ( 'NONE', #5585, 5.000000000000000888 ) ;
#11349=CYLINDRICAL_SURFACE ( 'NONE', #658, 15.00000000000000000 ) ;
#11350=VERTEX_POINT ( 'NONE', #3828 ) ;
#11353=EDGE_LOOP ( 'NONE', ( #2122, #4269, #6011 ) ) ;
#11359=CARTESIAN_POINT ( 'NONE',  ( 140.0000000000011369, 230.0000000000000853, -19.99999999999999645 ) ) ;
#11363=EDGE_CURVE ( 'NONE', #9072, #9665, #3173, .T. ) ;
#11375=DIRECTION ( 'NONE',  ( 1.564230817409691233E-15, 0.000000000000000000, -1.000000000000000000 ) ) ;
#11386=DIRECTION ( 'NONE',  ( -0.7071067811865447972, 0.7071067811865503483, 0.000000000000000000 ) ) ;
#11391=DIRECTION ( 'NONE',  ( -0.000000000000000000, -1.000000000000000000, -0.000000000000000000 ) ) ;
#11395=CARTESIAN_POINT ( 'NONE',  ( 71.59624044336383974, 44.46613403158139022, -22.48149205125841377 ) ) ;
#11398=CARTESIAN_POINT ( 'NONE',  ( -20.00000000000000355, 65.00000000000000000, -57.08203932499370836 ) ) ;
#11399=CARTESIAN_POINT ( 'NONE',  ( 71.05921646411502479, 17.18492608871972394, -24.19824146092191697 ) ) ;
#11401=DIRECTION ( 'NONE',  ( -1.000000000000000000, 8.326672684688666165E-15, 0.000000000000000000 ) ) ;
#11408=EDGE_CURVE ( 'NONE', #5372, #10506, #2256, .T. ) ;
#11412=ADVANCED_FACE ( 'NONE', ( #4889 ), #8677, .T. ) ;
#11414=CARTESIAN_POINT ( 'NONE',  ( 165.0000000000011369, 225.0000000000000853, 20.00000000000000000 ) ) ;
#11426=CARTESIAN_POINT ( 'NONE',  ( 71.75476781871510923, 49.45246612713112455, 21.82544253889693309 ) ) ;
#11429=CARTESIAN_POINT ( 'NONE',  ( 69.85318522031717237, 15.89659164372772970, 27.30472166927799194 ) ) ;
#11441=EDGE_CURVE ( 'NONE', #44, #12227, #4011, .T. ) ;
#11447=CARTESIAN_POINT ( 'NONE',  ( 4.953017525665607934, 43.69200144738164937, 74.83745130172235349 ) ) ;
#11448=VERTEX_POINT ( 'NONE', #5140 ) ;
#11452=DIRECTION ( 'NONE',  ( -0.000000000000000000, -1.000000000000000000, -0.000000000000000000 ) ) ;
#11456=PRESENTATION_STYLE_ASSIGNMENT (( #9624 ) ) ;
#11462=CARTESIAN_POINT ( 'NONE',  ( 77.45966692414833688, 50.00000000000008527, -20.00000000000000000 ) ) ;
#11464=CARTESIAN_POINT ( 'NONE',  ( 72.14031151490459592, 14.87472239508221072, -20.56889282981015654 ) ) ;
#11468=ADVANCED_FACE ( 'NONE', ( #8915 ), #10735, .T. ) ;
#11474=VERTEX_POINT ( 'NONE', #10678 ) ;
#11476=CARTESIAN_POINT ( 'NONE',  ( 74.16198487095665826, 40.00000000000009237, 25.00000000000000000 ) ) ;
#11477=ORIENTED_EDGE ( 'NONE', *, *, #2892, .T. ) ;
#11483=CYLINDRICAL_SURFACE ( 'NONE', #2894, 5.000000000000000888 ) ;
#11485=DIRECTION ( 'NONE',  ( -0.000000000000000000, -0.000000000000000000, -1.000000000000000000 ) ) ;
#11495=DIRECTION ( 'NONE',  ( 0.000000000000000000, -1.000000000000000000, 0.000000000000000000 ) ) ;
#11496=LINE ( 'NONE', #9539, #10859 ) ;
#11508=DIRECTION ( 'NONE',  ( -0.000000000000000000, -1.000000000000000000, -0.000000000000000000 ) ) ;
#11511=CARTESIAN_POINT ( 'NONE',  ( 0.000000000000000000, 65.00000000000000000, 0.000000000000000000 ) ) ;
#11520=CARTESIAN_POINT ( 'NONE',  ( 76.01088325117923716, 44.35544204059989681, -22.47665947743606907 ) ) ;
#11525=CARTESIAN_POINT ( 'NONE',  ( 76.01396467472481788, 15.64174653768074919, -22.47201498426100486 ) ) ;
#11539=CARTESIAN_POINT ( 'NONE',  ( 0.000000000000000000, -5.000000000000000000, 0.000000000000000000 ) ) ;
#11540=ORIENTED_EDGE ( 'NONE', *, *, #9498, .T. ) ;
#11543=AXIS2_PLACEMENT_3D ( 'NONE', #8747, #9869, #11823 ) ;
#11552=CARTESIAN_POINT ( 'NONE',  ( -14.00256363894252054, 22.13168096903907056, 73.68374432077325764 ) ) ;
#11556=ORIENTED_EDGE ( 'NONE', *, *, #6439, .T. ) ;
#11566=CIRCLE ( 'NONE', #814, 5.000000000000000888 ) ;
#11569=ORIENTED_EDGE ( 'NONE', *, *, #8475, .F. ) ;
#11571=CARTESIAN_POINT ( 'NONE',  ( 1.734723475976807094E-14, 65.00000000000000000, 57.08203932499370836 ) ) ;
#11575=FACE_OUTER_BOUND ( 'NONE', #6650, .T. ) ;
#11579=ORIENTED_EDGE ( 'NONE', *, *, #3947, .F. ) ;
#11589=CARTESIAN_POINT ( 'NONE',  ( 71.13616097333213872, 16.84684309240030231, -23.96252879557480497 ) ) ;
#11596=AXIS2_PLACEMENT_3D ( 'NONE', #10133, #9258, #12149 ) ;
#11601=DIRECTION ( 'NONE',  ( -1.000000000000000000, 0.000000000000000000, -0.000000000000000000 ) ) ;
#11605=ORIENTED_EDGE ( 'NONE', *, *, #4742, .F. ) ;
#11611=CARTESIAN_POINT ( 'NONE',  ( 150.0000000000010516, 15.00000000000008527, 22.92893218813452094 ) ) ;
#11616=DIRECTION ( 'NONE',  ( 1.000000000000000000, 0.000000000000000000, -1.224646799147353207E-16 ) ) ;
#11617=DIRECTION ( 'NONE',  ( 0.000000000000000000, 1.000000000000000000, -0.000000000000000000 ) ) ;
#11618=ORIENTED_EDGE ( 'NONE', *, *, #5216, .T. ) ;
#11622=CARTESIAN_POINT ( 'NONE',  ( 74.16198487095665826, 15.00000000000008882, 25.00000000000000000 ) ) ;
#11623=CARTESIAN_POINT ( 'NONE',  ( 0.000000000000000000, -10.00000000000000000, 70.00000000000001421 ) ) ;
#11633=CARTESIAN_POINT ( 'NONE',  ( 145.0000000000011369, 65.00000000000000000, 25.00000000000000000 ) ) ;
#11635=ORIENTED_EDGE ( 'NONE', *, *, #9007, .F. ) ;
#11640=CIRCLE ( 'NONE', #278, 15.00000000000000000 ) ;
#11643=EDGE_CURVE ( 'NONE', #9081, #11877, #6339, .T. ) ;
#11647=AXIS2_PLACEMENT_3D ( 'NONE', #4661, #3669, #11339 ) ;
#11649=CARTESIAN_POINT ( 'NONE',  ( 72.46134176498783575, 10.00000000076808249, -19.35843010035823397 ) ) ;
#11650=CARTESIAN_POINT ( 'NONE',  ( 71.66575360104040726, 10.66092814062295346, -22.11578253505649272 ) ) ;
#11651=DIRECTION ( 'NONE',  ( 0.000000000000000000, 0.000000000000000000, -1.000000000000000000 ) ) ;
#11658=ORIENTED_EDGE ( 'NONE', *, *, #1891, .F. ) ;
#11665=CARTESIAN_POINT ( 'NONE',  ( 140.0000000000011369, 225.0000000000000853, 20.00000000000000000 ) ) ;
#11671=AXIS2_PLACEMENT_3D ( 'NONE', #8542, #5004, #3008 ) ;
#11675=FACE_OUTER_BOUND ( 'NONE', #6954, .T. ) ;
#11676=EDGE_LOOP ( 'NONE', ( #1378, #9920, #1956 ) ) ;
#11683=LINE ( 'NONE', #4367, #6400 ) ;
#11684=VERTEX_POINT ( 'NONE', #11029 ) ;
#11695=DIRECTION ( 'NONE',  ( -0.000000000000000000, 1.000000000000000000, -0.000000000000000000 ) ) ;
#11699=LINE ( 'NONE', #10752, #7778 ) ;
#11702=ORIENTED_EDGE ( 'NONE', *, *, #7673, .T. ) ;
#11707=CARTESIAN_POINT ( 'NONE',  ( 70.67711243716091474, 12.63198440090825869, -25.09579365358156622 ) ) ;
#11728=EDGE_CURVE ( 'NONE', #11037, #6417, #8902, .T. ) ;
#11730=LINE ( 'NONE', #5068, #7469 ) ;
#11737=DIRECTION ( 'NONE',  ( 0.000000000000000000, 1.000000000000000000, 0.000000000000000000 ) ) ;
#11741=CARTESIAN_POINT ( 'NONE',  ( 69.72804008650275875, 16.70676746007779911, 27.62368211345550506 ) ) ;
#11746=EDGE_CURVE ( 'NONE', #9474, #10742, #12140, .T. ) ;
#11750=CARTESIAN_POINT ( 'NONE',  ( 74.37657609242708645, 41.64661626995485477, -24.73263046052358405 ) ) ;
#11753=DIRECTION ( 'NONE',  ( -0.000000000000000000, 0.000000000000000000, -1.000000000000000000 ) ) ;
#11754=CARTESIAN_POINT ( 'NONE',  ( 76.47662455941971871, 44.68978179728624411, 21.74119912861985071 ) ) ;
#11761=VERTEX_POINT ( 'NONE', #7479 ) ;
#11764=ORIENTED_EDGE ( 'NONE', *, *, #9281, .F. ) ;
#11767=EDGE_CURVE ( 'NONE', #5388, #10667, #11348, .T. ) ;
#11768=DIRECTION ( 'NONE',  ( 0.000000000000000000, 0.000000000000000000, -1.000000000000000000 ) ) ;
#11769=CARTESIAN_POINT ( 'NONE',  ( 77.45966692414835109, 10.00000000000008882, -19.99999999999999645 ) ) ;
#11771=CARTESIAN_POINT ( 'NONE',  ( 30.00000000000004263, 65.00000000000000000, -63.24555320336758513 ) ) ;
#11776=CARTESIAN_POINT ( 'NONE',  ( 0.000000000000000000, 10.00000000000017586, 0.000000000000000000 ) ) ;
#11788=ORIENTED_EDGE ( 'NONE', *, *, #1021, .T. ) ;
#11790=FACE_OUTER_BOUND ( 'NONE', #811, .T. ) ;
#11794=ORIENTED_EDGE ( 'NONE', *, *, #11746, .T. ) ;
#11795=CARTESIAN_POINT ( 'NONE',  ( 69.53296405455485285, 40.65417715541234855, -28.10992626845828113 ) ) ;
#11803=CARTESIAN_POINT ( 'NONE',  ( 70.88282142915605277, 12.08604768574887345, 24.51348554696365056 ) ) ;
#11804=EDGE_LOOP ( 'NONE', ( #11991, #7987, #9895, #958, #7999, #11000, #2782 ) ) ;
#11806=CARTESIAN_POINT ( 'NONE',  ( 76.23711339313383917, 44.53569103644999672, -22.12715364262389528 ) ) ;
#11807=PLANE ( 'NONE',  #8569 ) ;
#11810=CIRCLE ( 'NONE', #9999, 70.00000000000001421 ) ;
#11811=CARTESIAN_POINT ( 'NONE',  ( 72.28000013808933488, 14.83797322639769689, 20.04822706562307033 ) ) ;
#11814=CARTESIAN_POINT ( 'NONE',  ( 72.45961080413241007, 49.99999999876575885, -19.36513408292425709 ) ) ;
#11819=CARTESIAN_POINT ( 'NONE',  ( 70.86094439463602157, 41.47042339171561309, 24.79386831723889628 ) ) ;
#11823=DIRECTION ( 'NONE',  ( 0.000000000000000000, 0.000000000000000000, 1.000000000000000000 ) ) ;
#11830=DIRECTION ( 'NONE',  ( -1.000000000000000000, 0.000000000000000000, 0.000000000000000000 ) ) ;
#11831=DIRECTION ( 'NONE',  ( -0.000000000000000000, 1.000000000000000000, -0.000000000000000000 ) ) ;
#11834=PRODUCT_DEFINITION ( 'UNKNOWN', '', #5351, #2265 ) ;
#11835=VECTOR ( 'NONE', #9180, 1000.000000000000000 ) ;
#11837=DIRECTION ( 'NONE',  ( -0.000000000000000000, 1.000000000000000000, -0.000000000000000000 ) ) ;
#11849=CARTESIAN_POINT ( 'NONE',  ( 77.45966692414835109, 15.00000000000008882, -19.99999999999999645 ) ) ;
#11856=DIRECTION ( 'NONE',  ( 1.000000000000000000, -0.000000000000000000, 0.000000000000000000 ) ) ;
#11863=CYLINDRICAL_SURFACE ( 'NONE', #10372, 5.000000000000004441 ) ;
#11865=EDGE_LOOP ( 'NONE', ( #9351, #203, #2836, #4472 ) ) ;
#11871=CARTESIAN_POINT ( 'NONE',  ( 71.78384618016828256, 10.51296179634712580, 21.72949947218171118 ) ) ;
#11874=EDGE_LOOP ( 'NONE', ( #11259, #4740, #5768, #5072 ) ) ;
#11877=VERTEX_POINT ( 'NONE', #3672 ) ;
#11878=CYLINDRICAL_SURFACE ( 'NONE', #9824, 5.000000000000000888 ) ;
#11879=CARTESIAN_POINT ( 'NONE',  ( 71.31012073601122836, 43.75331323920969595, 23.41524959671097150 ) ) ;
#11880=EDGE_LOOP ( 'NONE', ( #3444, #9611, #9845, #11023 ) ) ;
#11887=ORIENTED_EDGE ( 'NONE', *, *, #2087, .T. ) ;
#11888=UNCERTAINTY_MEASURE_WITH_UNIT (LENGTH_MEASURE( 1.000000000000000082E-05 ), #9501, 'distance_accuracy_value', 'NONE');
#11890=LINE ( 'NONE', #1656, #11835 ) ;
#11892=ADVANCED_FACE ( 'NONE', ( #9391 ), #4664, .T. ) ;
#11894=DIRECTION ( 'NONE',  ( 0.000000000000000000, 0.000000000000000000, -1.000000000000000000 ) ) ;
#11895=CYLINDRICAL_SURFACE ( 'NONE', #11188, 3.399999999999999911 ) ;
#11900=CARTESIAN_POINT ( 'NONE',  ( 165.0000000000011369, 230.0000000000000853, -20.00000000000000000 ) ) ;
#11902=CARTESIAN_POINT ( 'NONE',  ( -30.00000000000004263, 65.00000000000000000, 57.08203932499370836 ) ) ;
#11906=ORIENTED_EDGE ( 'NONE', *, *, #405, .T. ) ;
#11907=DIRECTION ( 'NONE',  ( 0.000000000000000000, 0.000000000000000000, -1.000000000000000000 ) ) ;
#11913=CARTESIAN_POINT ( 'NONE',  ( 72.45442684796221045, 50.00000000000009237, -19.38521145883885666 ) ) ;
#11918=DIRECTION ( 'NONE',  ( 0.000000000000000000, 0.000000000000000000, 1.000000000000000000 ) ) ;
#11922=FACE_OUTER_BOUND ( 'NONE', #4421, .T. ) ;
#11929=ORIENTED_EDGE ( 'NONE', *, *, #8128, .F. ) ;
#11931=CARTESIAN_POINT ( 'NONE',  ( 75.73945001075399830, 15.90984549754468524, 22.88037593554966165 ) ) ;
#11934=CARTESIAN_POINT ( 'NONE',  ( 75.20175883194669098, 16.56455603843833657, 23.64678730934253537 ) ) ;
#11938=CARTESIAN_POINT ( 'NONE',  ( 74.58021194344081550, 42.25882445080058147, 24.47298709600845612 ) ) ;
#11945=EDGE_CURVE ( 'NONE', #4047, #4313, #6184, .T. ) ;
#11955=CARTESIAN_POINT ( 'NONE',  ( 69.76162866618028602, 16.50146430099879780, -27.53780242413600732 ) ) ;
#11963=CIRCLE ( 'NONE', #6585, 5.000000000000001776 ) ;
#11967=CARTESIAN_POINT ( 'NONE',  ( 77.45966692414835109, 45.00000000000008527, -20.00000000000000000 ) ) ;
#11968=CARTESIAN_POINT ( 'NONE',  ( 75.70364277637115435, 15.94008215020948427, -22.93512150616605183 ) ) ;
#11971=DIRECTION ( 'NONE',  ( 0.000000000000000000, -1.000000000000000000, 0.000000000000000000 ) ) ;
#11980=CIRCLE ( 'NONE', #7396, 15.00000000000000000 ) ;
#11986=CARTESIAN_POINT ( 'NONE',  ( 71.22480170918207421, 11.35480001874193690, 23.50133972577969743 ) ) ;
#11991=ORIENTED_EDGE ( 'NONE', *, *, #4636, .F. ) ;
#11993=CARTESIAN_POINT ( 'NONE',  ( 70.44139041661959766, 13.32009519262272690, 25.75312943552223643 ) ) ;
#11995=ORIENTED_EDGE ( 'NONE', *, *, #12299, .F. ) ;
#12000=CARTESIAN_POINT ( 'NONE',  ( 76.19870213673728188, 44.50753802327100317, 22.18755841417295827 ) ) ;
#12001=EDGE_LOOP ( 'NONE', ( #8891, #10076, #5243, #4407 ) ) ;
#12011=CARTESIAN_POINT ( 'NONE',  ( 165.0000000000011369, 37.07106781186552524, -25.00000000000000000 ) ) ;
#12028=DIRECTION ( 'NONE',  ( 0.000000000000000000, 0.000000000000000000, 1.000000000000000000 ) ) ;
#12035=ORIENTED_EDGE ( 'NONE', *, *, #10642, .T. ) ;
#12050=DIRECTION ( 'NONE',  ( -0.000000000000000000, 1.000000000000000000, 0.000000000000000000 ) ) ;
#12063=DIRECTION ( 'NONE',  ( 0.000000000000000000, 0.000000000000000000, 1.000000000000000000 ) ) ;
#12069=ORIENTED_EDGE ( 'NONE', *, *, #2721, .F. ) ;
#12083=CARTESIAN_POINT ( 'NONE',  ( 0.000000000000000000, 75.00000000000000000, 25.00000000000000000 ) ) ;
#12084=CARTESIAN_POINT ( 'NONE',  ( 13.78766650650841186, 29.07005748252881361, 73.72178925532224980 ) ) ;
#12088=DIRECTION ( 'NONE',  ( -0.000000000000000000, 1.000000000000000000, -0.000000000000000000 ) ) ;
#12090=CARTESIAN_POINT ( 'NONE',  ( 0.000000000000000000, 10.00000000000017586, 75.00000000000001421 ) ) ;
#12094=DIRECTION ( 'NONE',  ( 0.000000000000000000, 0.000000000000000000, 1.000000000000000000 ) ) ;
#12095=ORIENTED_EDGE ( 'NONE', *, *, #3285, .F. ) ;
#12098=CARTESIAN_POINT ( 'NONE',  ( 0.000000000000000000, 15.00000000000008882, 0.000000000000000000 ) ) ;
#12105=CARTESIAN_POINT ( 'NONE',  ( 117.9289321881355193, 40.00000000000009237, -20.00000000000000000 ) ) ;
#12122=CARTESIAN_POINT ( 'NONE',  ( 70.88057259133860555, 47.89215595910781786, 24.51542725512078746 ) ) ;
#12123=ORIENTED_EDGE ( 'NONE', *, *, #3925, .F. ) ;
#12126=ORIENTED_EDGE ( 'NONE', *, *, #4197, .T. ) ;
#12132=ORIENTED_EDGE ( 'NONE', *, *, #12299, .T. ) ;
#12134=EDGE_CURVE ( 'NONE', #9665, #8933, #7385, .T. ) ;
#12139=DIRECTION ( 'NONE',  ( 0.000000000000000000, 0.000000000000000000, -1.000000000000000000 ) ) ;
#12140=B_SPLINE_CURVE_WITH_KNOTS ( 'NONE', 3,
 ( #6296, #6235, #11795, #1560, #10966, #3369, #3240, #7042, #5362, #10841, #2303, #6114, #1373, #8027, #5241, #555, #10903, #9019, #3435, #495, #10025, #8091, #11913, #4352 ),
 .UNSPECIFIED., .F., .F.,
 ( 4, 2, 2, 2, 2, 2, 2, 2, 2, 2, 2, 4 ),
 ( 0.000000000000000000, 0.0009796746052620941732, 0.001959349210524188346, 0.003918698421048397509, 0.004898373026310511198, 0.005878047631572623152, 0.007837396842096862673, 0.009796746052621102194, 0.01175609526314533824, 0.01273576986840745454, 0.01371544447366956909, 0.01567479368419381555 ),
 .UNSPECIFIED. ) ;
#12149=DIRECTION ( 'NONE',  ( 0.000000000000000000, 0.000000000000000000, -1.000000000000000000 ) ) ;
#12153=FACE_OUTER_BOUND ( 'NONE', #9276, .T. ) ;
#12163=EDGE_LOOP ( 'NONE', ( #11060, #3863, #7053, #2380, #8604, #6519 ) ) ;
#12167=EDGE_LOOP ( 'NONE', ( #11995, #9874, #5139, #8957 ) ) ;
#12168=DIRECTION ( 'NONE',  ( 0.9682458365518540333, 0.000000000000000000, -0.2500000000000003331 ) ) ;
#12173=VECTOR ( 'NONE', #5153, 999.9999999999998863 ) ;
#12176=ORIENTED_EDGE ( 'NONE', *, *, #9647, .T. ) ;
#12179=CARTESIAN_POINT ( 'NONE',  ( 70.79098555864042908, 20.00000000000009237, 25.00000000000000000 ) ) ;
#12185=CARTESIAN_POINT ( 'NONE',  ( 70.26686370603786713, 46.04793283185657060, 26.22231631056804346 ) ) ;
#12195=PLANE ( 'NONE',  #11068 ) ;
#12202=DIRECTION ( 'NONE',  ( -1.000000000000000000, 0.000000000000000000, 0.000000000000000000 ) ) ;
#12207=EDGE_CURVE ( 'NONE', #10533, #1040, #11963, .T. ) ;
#12227=VERTEX_POINT ( 'NONE', #1731 ) ;
#12228=EDGE_LOOP ( 'NONE', ( #9452, #9456, #2315, #2798 ) ) ;
#12233=DIRECTION ( 'NONE',  ( 1.000000000000000000, 0.000000000000000000, -3.469446951953613696E-16 ) ) ;
#12237=AXIS2_PLACEMENT_3D ( 'NONE', #552, #2358, #4349 ) ;
#12242=DIRECTION ( 'NONE',  ( -1.000000000000000000, 0.000000000000000000, 0.000000000000000000 ) ) ;
#12243=CARTESIAN_POINT ( 'NONE',  ( -15.63313230619844241, 25.91538294882372995, 73.35278444408292842 ) ) ;
#12247=FACE_OUTER_BOUND ( 'NONE', #11173, .T. ) ;
#12248=LINE ( 'NONE', #6445, #1316 ) ;
#12254=CIRCLE ( 'NONE', #905, 75.00000000000001421 ) ;
#12268=VECTOR ( 'NONE', #10976, 1000.000000000000000 ) ;
#12269=EDGE_CURVE ( 'NONE', #2354, #1231, #11082, .T. ) ;
#12270=FACE_OUTER_BOUND ( 'NONE', #12163, .T. ) ;
#12273=ORIENTED_EDGE ( 'NONE', *, *, #4742, .T. ) ;
#12276=CARTESIAN_POINT ( 'NONE',  ( 70.80917463421377533, 19.14431278602349096, -24.94686153084484204 ) ) ;
#12299=EDGE_CURVE ( 'NONE', #712, #5882, #7519, .T. ) ;
#12303=CARTESIAN_POINT ( 'NONE',  ( 72.45461974811382788, 50.00000000000007105, 19.38446435976420190 ) ) ;
#12304=ORIENTED_EDGE ( 'NONE', *, *, #5007, .T. ) ;
#12306=CARTESIAN_POINT ( 'NONE',  ( 72.46134176498804891, 49.99999999923035432, 19.35843010035742040 ) ) ;
#12321=CARTESIAN_POINT ( 'NONE',  ( -20.00000000000000355, 63.00000000000000000, -57.08203932499370836 ) ) ;
#12327=SURFACE_SIDE_STYLE ('',( #2969 ) ) ;
#12330=CARTESIAN_POINT ( 'NONE',  ( 70.79098555865897424, 40.21264271670013102, -24.99999999997160316 ) ) ;
#12331=FACE_OUTER_BOUND ( 'NONE', #8036, .T. ) ;
#12335=CARTESIAN_POINT ( 'NONE',  ( 165.0000000000011369, 0.000000000000000000, 25.00000000000000000 ) ) ;
#12336=ORIENTED_EDGE ( 'NONE', *, *, #10028, .T. ) ;
#12339=CIRCLE ( 'NONE', #4167, 5.000000000000000888 ) ;
#12348=CARTESIAN_POINT ( 'NONE',  ( 20.00000000000000355, 50.00000000000000000, 57.08203932499370836 ) ) ;
ENDSEC;
END-ISO-10303-21;
